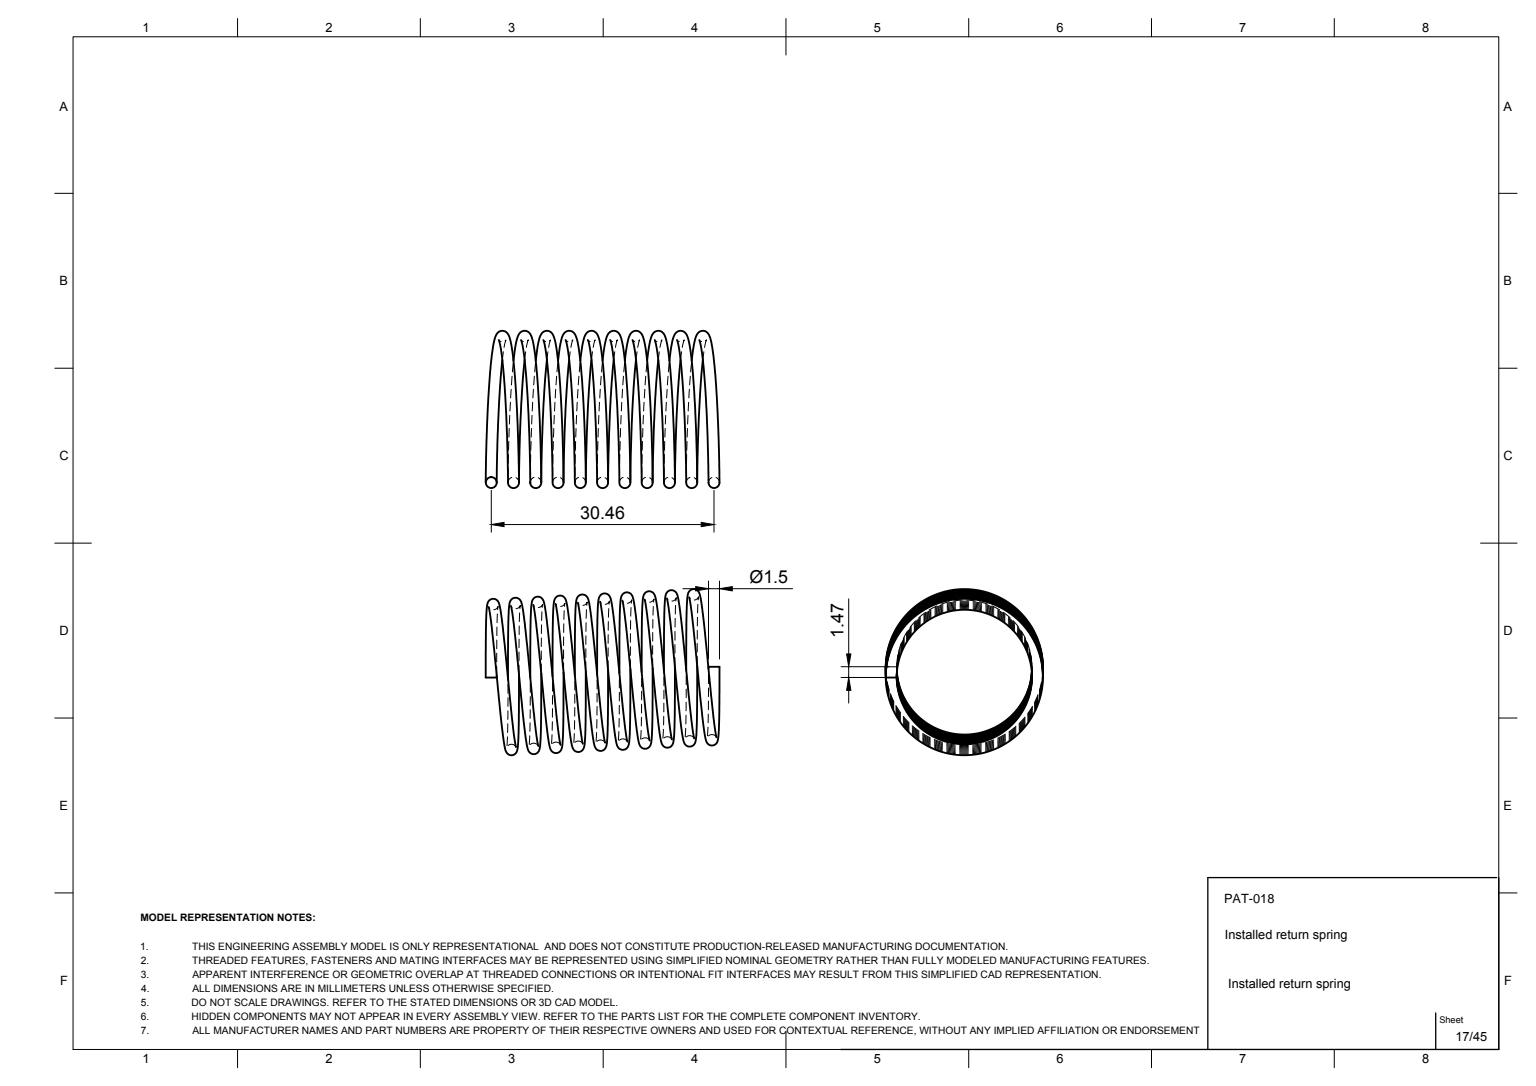
ISO-10303-21;
HEADER;
/* Generated by software containing ST-Developer
 * from STEP Tools, Inc. (www.steptools.com) 
 */

FILE_DESCRIPTION(
/* description */ ('Cam-driven reciprocating slide'),
/* implementation_level */ '2;1');

FILE_NAME(
/* name */ 'Installed return spring.step',
/* time_stamp */ '2026-10-28T03:25:20-07:00',
/* author */ (''),
/* organization */ (''),
/* preprocessor_version */ 'ST-DEVELOPER v20.2',
/* originating_system */ 'Autodesk Translation Framework v15.17.0.0',
/* authorisation */ '');

FILE_SCHEMA (('AUTOMOTIVE_DESIGN { 1 0 10303 214 3 1 1 }'));
ENDSEC;

DATA;
#10=MECHANICAL_DESIGN_GEOMETRIC_PRESENTATION_REPRESENTATION('',(#434),#13277);
#332=B_SPLINE_CURVE_WITH_KNOTS('',3,(#11701,#11702,#11703,#11704,#11705,
#11706,#11707,#11708,#11709,#11710,#11711,#11712,#11713,#11714,#11715,#11716,
#11717,#11718,#11719,#11720,#11721,#11722,#11723,#11724,#11725,#11726,#11727,
#11728,#11729,#11730,#11731,#11732,#11733,#11734,#11735,#11736,#11737,#11738,
#11739,#11740,#11741,#11742,#11743,#11744,#11745,#11746,#11747,#11748,#11749,
#11750,#11751,#11752,#11753,#11754,#11755,#11756,#11757,#11758,#11759,#11760,
#11761,#11762,#11763,#11764,#11765,#11766,#11767,#11768,#11769,#11770,#11771,
#11772,#11773,#11774,#11775,#11776,#11777,#11778,#11779,#11780,#11781,#11782,
#11783,#11784,#11785,#11786,#11787,#11788,#11789,#11790,#11791,#11792,#11793,
#11794,#11795,#11796,#11797,#11798,#11799,#11800,#11801,#11802,#11803,#11804,
#11805,#11806,#11807,#11808,#11809,#11810,#11811,#11812,#11813,#11814,#11815,
#11816,#11817,#11818,#11819,#11820,#11821,#11822,#11823,#11824),
 .UNSPECIFIED.,.F.,.F.,(4,1,1,1,1,1,1,1,1,1,1,1,1,1,1,1,1,1,1,1,1,1,1,1,
1,1,1,1,1,1,1,1,1,1,1,1,1,1,1,1,1,1,1,1,1,1,1,1,1,1,1,1,1,1,1,1,1,1,1,1,
1,1,1,1,1,1,1,1,1,1,1,1,1,1,1,1,1,1,1,1,1,1,1,1,1,1,1,1,1,1,1,1,1,1,1,1,
1,1,1,1,1,1,1,1,1,1,1,1,1,1,1,1,1,1,1,1,1,1,1,1,1,4),(0.,0.00892857142857143,
0.0178571428571429,0.0267857142857143,0.0357142857142857,0.0446428571428571,
0.0535714285714286,0.0625,0.0714285714285714,0.0803571428571428,0.0892857142857143,
0.0982142857142857,0.107142857142857,0.116071428571429,0.125,0.133928571428571,
0.142857142857143,0.150793650793651,0.154761904761905,0.156746031746032,
0.158730158730159,0.166666666666667,0.174603174603175,0.182539682539683,
0.19047619047619,0.202380952380952,0.214285714285714,0.222222222222222,
0.23015873015873,0.238095238095238,0.244047619047619,0.25,0.261904761904762,
0.273809523809524,0.285714285714286,0.297619047619048,0.30952380952381,
0.321428571428571,0.327380952380952,0.333333333333333,0.341269841269841,
0.349206349206349,0.357142857142857,0.365079365079365,0.373015873015873,
0.380952380952381,0.386904761904762,0.392857142857143,0.404761904761905,
0.416666666666667,0.422619047619048,0.428571428571429,0.4375,0.446428571428571,
0.455357142857143,0.464285714285714,0.468253968253968,0.476190476190476,
0.482142857142857,0.488095238095238,0.494047619047619,0.5,0.504464285714286,
0.508928571428571,0.517857142857143,0.526785714285714,0.535714285714286,
0.540178571428571,0.544642857142857,0.553571428571429,0.5625,0.571428571428571,
0.580357142857143,0.589285714285714,0.598214285714286,0.607142857142857,
0.616071428571429,0.625,0.633928571428571,0.642857142857143,0.650793650793651,
0.658730158730159,0.666666666666667,0.672619047619048,0.678571428571428,
0.69047619047619,0.696428571428571,0.702380952380952,0.714285714285714,
0.726190476190476,0.738095238095238,0.746031746031746,0.753968253968254,
0.761904761904762,0.76984126984127,0.777777777777778,0.785714285714286,
0.790178571428571,0.794642857142857,0.803571428571428,0.8125,0.821428571428571,
0.830357142857143,0.839285714285714,0.848214285714286,0.857142857142857,
0.866071428571429,0.875,0.883928571428571,0.892857142857143,0.901785714285714,
0.910714285714286,0.919642857142857,0.928571428571429,0.9375,0.946428571428571,
0.955357142857143,0.964285714285714,0.973214285714286,0.982142857142857,
0.991071428571429,1.),.UNSPECIFIED.);
#347=B_SPLINE_SURFACE_WITH_KNOTS('',3,3,((#10458,#10459,#10460,#10461,#10462,
#10463,#10464,#10465,#10466,#10467,#10468,#10469,#10470,#10471,#10472,#10473,
#10474,#10475,#10476,#10477,#10478,#10479,#10480,#10481,#10482,#10483,#10484,
#10485,#10486,#10487,#10488,#10489,#10490,#10491,#10492,#10493,#10494,#10495,
#10496,#10497,#10498,#10499,#10500,#10501,#10502,#10503,#10504,#10505,#10506,
#10507,#10508,#10509,#10510,#10511,#10512,#10513,#10514,#10515,#10516,#10517,
#10518,#10519,#10520,#10521,#10522,#10523,#10524,#10525,#10526,#10527,#10528,
#10529,#10530,#10531,#10532,#10533,#10534,#10535,#10536,#10537,#10538,#10539,
#10540,#10541,#10542,#10543,#10544,#10545,#10546,#10547,#10548,#10549,#10550,
#10551,#10552,#10553,#10554,#10555,#10556,#10557,#10558,#10559,#10560,#10561,
#10562,#10563,#10564,#10565,#10566,#10567,#10568,#10569,#10570,#10571,#10572,
#10573,#10574,#10575,#10576,#10577,#10578,#10579,#10580,#10581),(#10582,
#10583,#10584,#10585,#10586,#10587,#10588,#10589,#10590,#10591,#10592,#10593,
#10594,#10595,#10596,#10597,#10598,#10599,#10600,#10601,#10602,#10603,#10604,
#10605,#10606,#10607,#10608,#10609,#10610,#10611,#10612,#10613,#10614,#10615,
#10616,#10617,#10618,#10619,#10620,#10621,#10622,#10623,#10624,#10625,#10626,
#10627,#10628,#10629,#10630,#10631,#10632,#10633,#10634,#10635,#10636,#10637,
#10638,#10639,#10640,#10641,#10642,#10643,#10644,#10645,#10646,#10647,#10648,
#10649,#10650,#10651,#10652,#10653,#10654,#10655,#10656,#10657,#10658,#10659,
#10660,#10661,#10662,#10663,#10664,#10665,#10666,#10667,#10668,#10669,#10670,
#10671,#10672,#10673,#10674,#10675,#10676,#10677,#10678,#10679,#10680,#10681,
#10682,#10683,#10684,#10685,#10686,#10687,#10688,#10689,#10690,#10691,#10692,
#10693,#10694,#10695,#10696,#10697,#10698,#10699,#10700,#10701,#10702,#10703,
#10704,#10705),(#10706,#10707,#10708,#10709,#10710,#10711,#10712,#10713,
#10714,#10715,#10716,#10717,#10718,#10719,#10720,#10721,#10722,#10723,#10724,
#10725,#10726,#10727,#10728,#10729,#10730,#10731,#10732,#10733,#10734,#10735,
#10736,#10737,#10738,#10739,#10740,#10741,#10742,#10743,#10744,#10745,#10746,
#10747,#10748,#10749,#10750,#10751,#10752,#10753,#10754,#10755,#10756,#10757,
#10758,#10759,#10760,#10761,#10762,#10763,#10764,#10765,#10766,#10767,#10768,
#10769,#10770,#10771,#10772,#10773,#10774,#10775,#10776,#10777,#10778,#10779,
#10780,#10781,#10782,#10783,#10784,#10785,#10786,#10787,#10788,#10789,#10790,
#10791,#10792,#10793,#10794,#10795,#10796,#10797,#10798,#10799,#10800,#10801,
#10802,#10803,#10804,#10805,#10806,#10807,#10808,#10809,#10810,#10811,#10812,
#10813,#10814,#10815,#10816,#10817,#10818,#10819,#10820,#10821,#10822,#10823,
#10824,#10825,#10826,#10827,#10828,#10829),(#10830,#10831,#10832,#10833,
#10834,#10835,#10836,#10837,#10838,#10839,#10840,#10841,#10842,#10843,#10844,
#10845,#10846,#10847,#10848,#10849,#10850,#10851,#10852,#10853,#10854,#10855,
#10856,#10857,#10858,#10859,#10860,#10861,#10862,#10863,#10864,#10865,#10866,
#10867,#10868,#10869,#10870,#10871,#10872,#10873,#10874,#10875,#10876,#10877,
#10878,#10879,#10880,#10881,#10882,#10883,#10884,#10885,#10886,#10887,#10888,
#10889,#10890,#10891,#10892,#10893,#10894,#10895,#10896,#10897,#10898,#10899,
#10900,#10901,#10902,#10903,#10904,#10905,#10906,#10907,#10908,#10909,#10910,
#10911,#10912,#10913,#10914,#10915,#10916,#10917,#10918,#10919,#10920,#10921,
#10922,#10923,#10924,#10925,#10926,#10927,#10928,#10929,#10930,#10931,#10932,
#10933,#10934,#10935,#10936,#10937,#10938,#10939,#10940,#10941,#10942,#10943,
#10944,#10945,#10946,#10947,#10948,#10949,#10950,#10951,#10952,#10953),
(#10954,#10955,#10956,#10957,#10958,#10959,#10960,#10961,#10962,#10963,
#10964,#10965,#10966,#10967,#10968,#10969,#10970,#10971,#10972,#10973,#10974,
#10975,#10976,#10977,#10978,#10979,#10980,#10981,#10982,#10983,#10984,#10985,
#10986,#10987,#10988,#10989,#10990,#10991,#10992,#10993,#10994,#10995,#10996,
#10997,#10998,#10999,#11000,#11001,#11002,#11003,#11004,#11005,#11006,#11007,
#11008,#11009,#11010,#11011,#11012,#11013,#11014,#11015,#11016,#11017,#11018,
#11019,#11020,#11021,#11022,#11023,#11024,#11025,#11026,#11027,#11028,#11029,
#11030,#11031,#11032,#11033,#11034,#11035,#11036,#11037,#11038,#11039,#11040,
#11041,#11042,#11043,#11044,#11045,#11046,#11047,#11048,#11049,#11050,#11051,
#11052,#11053,#11054,#11055,#11056,#11057,#11058,#11059,#11060,#11061,#11062,
#11063,#11064,#11065,#11066,#11067,#11068,#11069,#11070,#11071,#11072,#11073,
#11074,#11075,#11076,#11077),(#11078,#11079,#11080,#11081,#11082,#11083,
#11084,#11085,#11086,#11087,#11088,#11089,#11090,#11091,#11092,#11093,#11094,
#11095,#11096,#11097,#11098,#11099,#11100,#11101,#11102,#11103,#11104,#11105,
#11106,#11107,#11108,#11109,#11110,#11111,#11112,#11113,#11114,#11115,#11116,
#11117,#11118,#11119,#11120,#11121,#11122,#11123,#11124,#11125,#11126,#11127,
#11128,#11129,#11130,#11131,#11132,#11133,#11134,#11135,#11136,#11137,#11138,
#11139,#11140,#11141,#11142,#11143,#11144,#11145,#11146,#11147,#11148,#11149,
#11150,#11151,#11152,#11153,#11154,#11155,#11156,#11157,#11158,#11159,#11160,
#11161,#11162,#11163,#11164,#11165,#11166,#11167,#11168,#11169,#11170,#11171,
#11172,#11173,#11174,#11175,#11176,#11177,#11178,#11179,#11180,#11181,#11182,
#11183,#11184,#11185,#11186,#11187,#11188,#11189,#11190,#11191,#11192,#11193,
#11194,#11195,#11196,#11197,#11198,#11199,#11200,#11201),(#11202,#11203,
#11204,#11205,#11206,#11207,#11208,#11209,#11210,#11211,#11212,#11213,#11214,
#11215,#11216,#11217,#11218,#11219,#11220,#11221,#11222,#11223,#11224,#11225,
#11226,#11227,#11228,#11229,#11230,#11231,#11232,#11233,#11234,#11235,#11236,
#11237,#11238,#11239,#11240,#11241,#11242,#11243,#11244,#11245,#11246,#11247,
#11248,#11249,#11250,#11251,#11252,#11253,#11254,#11255,#11256,#11257,#11258,
#11259,#11260,#11261,#11262,#11263,#11264,#11265,#11266,#11267,#11268,#11269,
#11270,#11271,#11272,#11273,#11274,#11275,#11276,#11277,#11278,#11279,#11280,
#11281,#11282,#11283,#11284,#11285,#11286,#11287,#11288,#11289,#11290,#11291,
#11292,#11293,#11294,#11295,#11296,#11297,#11298,#11299,#11300,#11301,#11302,
#11303,#11304,#11305,#11306,#11307,#11308,#11309,#11310,#11311,#11312,#11313,
#11314,#11315,#11316,#11317,#11318,#11319,#11320,#11321,#11322,#11323,#11324,
#11325),(#11326,#11327,#11328,#11329,#11330,#11331,#11332,#11333,#11334,
#11335,#11336,#11337,#11338,#11339,#11340,#11341,#11342,#11343,#11344,#11345,
#11346,#11347,#11348,#11349,#11350,#11351,#11352,#11353,#11354,#11355,#11356,
#11357,#11358,#11359,#11360,#11361,#11362,#11363,#11364,#11365,#11366,#11367,
#11368,#11369,#11370,#11371,#11372,#11373,#11374,#11375,#11376,#11377,#11378,
#11379,#11380,#11381,#11382,#11383,#11384,#11385,#11386,#11387,#11388,#11389,
#11390,#11391,#11392,#11393,#11394,#11395,#11396,#11397,#11398,#11399,#11400,
#11401,#11402,#11403,#11404,#11405,#11406,#11407,#11408,#11409,#11410,#11411,
#11412,#11413,#11414,#11415,#11416,#11417,#11418,#11419,#11420,#11421,#11422,
#11423,#11424,#11425,#11426,#11427,#11428,#11429,#11430,#11431,#11432,#11433,
#11434,#11435,#11436,#11437,#11438,#11439,#11440,#11441,#11442,#11443,#11444,
#11445,#11446,#11447,#11448,#11449),(#11450,#11451,#11452,#11453,#11454,
#11455,#11456,#11457,#11458,#11459,#11460,#11461,#11462,#11463,#11464,#11465,
#11466,#11467,#11468,#11469,#11470,#11471,#11472,#11473,#11474,#11475,#11476,
#11477,#11478,#11479,#11480,#11481,#11482,#11483,#11484,#11485,#11486,#11487,
#11488,#11489,#11490,#11491,#11492,#11493,#11494,#11495,#11496,#11497,#11498,
#11499,#11500,#11501,#11502,#11503,#11504,#11505,#11506,#11507,#11508,#11509,
#11510,#11511,#11512,#11513,#11514,#11515,#11516,#11517,#11518,#11519,#11520,
#11521,#11522,#11523,#11524,#11525,#11526,#11527,#11528,#11529,#11530,#11531,
#11532,#11533,#11534,#11535,#11536,#11537,#11538,#11539,#11540,#11541,#11542,
#11543,#11544,#11545,#11546,#11547,#11548,#11549,#11550,#11551,#11552,#11553,
#11554,#11555,#11556,#11557,#11558,#11559,#11560,#11561,#11562,#11563,#11564,
#11565,#11566,#11567,#11568,#11569,#11570,#11571,#11572,#11573),(#11574,
#11575,#11576,#11577,#11578,#11579,#11580,#11581,#11582,#11583,#11584,#11585,
#11586,#11587,#11588,#11589,#11590,#11591,#11592,#11593,#11594,#11595,#11596,
#11597,#11598,#11599,#11600,#11601,#11602,#11603,#11604,#11605,#11606,#11607,
#11608,#11609,#11610,#11611,#11612,#11613,#11614,#11615,#11616,#11617,#11618,
#11619,#11620,#11621,#11622,#11623,#11624,#11625,#11626,#11627,#11628,#11629,
#11630,#11631,#11632,#11633,#11634,#11635,#11636,#11637,#11638,#11639,#11640,
#11641,#11642,#11643,#11644,#11645,#11646,#11647,#11648,#11649,#11650,#11651,
#11652,#11653,#11654,#11655,#11656,#11657,#11658,#11659,#11660,#11661,#11662,
#11663,#11664,#11665,#11666,#11667,#11668,#11669,#11670,#11671,#11672,#11673,
#11674,#11675,#11676,#11677,#11678,#11679,#11680,#11681,#11682,#11683,#11684,
#11685,#11686,#11687,#11688,#11689,#11690,#11691,#11692,#11693,#11694,#11695,
#11696,#11697)),.UNSPECIFIED.,.T.,.F.,.F.,(4,1,1,1,1,1,1,4),(4,1,1,1,1,
1,1,1,1,1,1,1,1,1,1,1,1,1,1,1,1,1,1,1,1,1,1,1,1,1,1,1,1,1,1,1,1,1,1,1,1,
1,1,1,1,1,1,1,1,1,1,1,1,1,1,1,1,1,1,1,1,1,1,1,1,1,1,1,1,1,1,1,1,1,1,1,1,
1,1,1,1,1,1,1,1,1,1,1,1,1,1,1,1,1,1,1,1,1,1,1,1,1,1,1,1,1,1,1,1,1,1,1,1,
1,1,1,1,1,1,1,1,4),(-3.14159265358979,-2.24399475256414,-1.34639685153848,
-0.448798950512828,0.448798950512828,1.34639685153848,2.24399475256414,
3.14159265358979),(0.,0.00892857142857143,0.0178571428571429,0.0267857142857143,
0.0357142857142857,0.0446428571428571,0.0535714285714286,0.0625,0.0714285714285714,
0.0803571428571428,0.0892857142857143,0.0982142857142857,0.107142857142857,
0.116071428571429,0.125,0.133928571428571,0.142857142857143,0.150793650793651,
0.154761904761905,0.156746031746032,0.158730158730159,0.166666666666667,
0.174603174603175,0.182539682539683,0.19047619047619,0.202380952380952,
0.214285714285714,0.222222222222222,0.23015873015873,0.238095238095238,
0.244047619047619,0.25,0.261904761904762,0.273809523809524,0.285714285714286,
0.297619047619048,0.30952380952381,0.321428571428571,0.327380952380952,
0.333333333333333,0.341269841269841,0.349206349206349,0.357142857142857,
0.365079365079365,0.373015873015873,0.380952380952381,0.386904761904762,
0.392857142857143,0.404761904761905,0.416666666666667,0.422619047619048,
0.428571428571429,0.4375,0.446428571428571,0.455357142857143,0.464285714285714,
0.468253968253968,0.476190476190476,0.482142857142857,0.488095238095238,
0.494047619047619,0.5,0.504464285714286,0.508928571428571,0.517857142857143,
0.526785714285714,0.535714285714286,0.540178571428571,0.544642857142857,
0.553571428571429,0.5625,0.571428571428571,0.580357142857143,0.589285714285714,
0.598214285714286,0.607142857142857,0.616071428571429,0.625,0.633928571428571,
0.642857142857143,0.650793650793651,0.658730158730159,0.666666666666667,
0.672619047619048,0.678571428571428,0.69047619047619,0.696428571428571,
0.702380952380952,0.714285714285714,0.726190476190476,0.738095238095238,
0.746031746031746,0.753968253968254,0.761904761904762,0.76984126984127,
0.777777777777778,0.785714285714286,0.790178571428571,0.794642857142857,
0.803571428571428,0.8125,0.821428571428571,0.830357142857143,0.839285714285714,
0.848214285714286,0.857142857142857,0.866071428571429,0.875,0.883928571428571,
0.892857142857143,0.901785714285714,0.910714285714286,0.919642857142857,
0.928571428571429,0.9375,0.946428571428571,0.955357142857143,0.964285714285714,
0.973214285714286,0.982142857142857,0.991071428571429,1.),.UNSPECIFIED.);
#360=SHAPE_REPRESENTATION_RELATIONSHIP('SRR','None',#13453,#397);
#397=ADVANCED_BREP_SHAPE_REPRESENTATION('',(#478),#13248);
#434=STYLED_ITEM('',(#13720),#478);
#478=MANIFOLD_SOLID_BREP('Body1',#6410);
#762=PLANE('',#7152);
#763=PLANE('',#7153);
#1049=FACE_OUTER_BOUND('',#1539,.T.);
#1050=FACE_OUTER_BOUND('',#1540,.T.);
#1051=FACE_OUTER_BOUND('',#1541,.T.);
#1539=EDGE_LOOP('',(#5002,#5003,#5004,#5005));
#1540=EDGE_LOOP('',(#5006));
#1541=EDGE_LOOP('',(#5007));
#2845=CIRCLE('',#7150,0.075);
#2846=CIRCLE('',#7151,0.075);
#3257=VERTEX_POINT('',#11698);
#3258=VERTEX_POINT('',#11700);
#3891=EDGE_CURVE('',#3257,#3257,#2845,.T.);
#3892=EDGE_CURVE('',#3257,#3258,#332,.T.);
#3893=EDGE_CURVE('',#3258,#3258,#2846,.T.);
#5002=ORIENTED_EDGE('',*,*,#3891,.T.);
#5003=ORIENTED_EDGE('',*,*,#3892,.T.);
#5004=ORIENTED_EDGE('',*,*,#3893,.F.);
#5005=ORIENTED_EDGE('',*,*,#3892,.F.);
#5006=ORIENTED_EDGE('',*,*,#3893,.T.);
#5007=ORIENTED_EDGE('',*,*,#3891,.F.);
#6167=ADVANCED_FACE('',(#1049),#347,.T.);
#6168=ADVANCED_FACE('',(#1050),#762,.T.);
#6169=ADVANCED_FACE('',(#1051),#763,.F.);
#6410=CLOSED_SHELL('',(#6167,#6168,#6169));
#7149=AXIS2_PLACEMENT_3D('',#10457,#8460,#8461);
#7150=AXIS2_PLACEMENT_3D('',#11699,#8462,#8463);
#7151=AXIS2_PLACEMENT_3D('',#11825,#8464,#8465);
#7152=AXIS2_PLACEMENT_3D('',#11826,#8466,#8467);
#7153=AXIS2_PLACEMENT_3D('',#11827,#8468,#8469);
#8460=DIRECTION('axis',(0.,0.,1.));
#8461=DIRECTION('refdir',(1.,0.,0.));
#8462=DIRECTION('center_axis',(-0.000134463754131944,0.998830887797922,
0.0483408678067963));
#8463=DIRECTION('ref_axis',(6.50770273904549E-6,-0.0483408673687592,0.998830896848754));
#8464=DIRECTION('center_axis',(0.000134463742439319,0.998830887795465,0.0483408678575998));
#8465=DIRECTION('ref_axis',(-0.0950425701692232,0.0481348041224881,-0.994308780252753));
#8466=DIRECTION('center_axis',(0.000134463742439319,0.998830887795465,0.0483408678575998));
#8467=DIRECTION('ref_axis',(-0.0950425701692232,0.0481348041224881,-0.994308780252753));
#8468=DIRECTION('center_axis',(-0.000134463754131944,0.998830887797922,
0.0483408678067963));
#8469=DIRECTION('ref_axis',(6.50770273904549E-6,-0.0483408673687592,0.998830896848754));
#10457=CARTESIAN_POINT('',(0.,0.,0.));
#10458=CARTESIAN_POINT('Ctrl Pts',(0.999999511922295,0.00362556505265694,
7.80008768273634));
#10459=CARTESIAN_POINT('Ctrl Pts',(0.999974254701651,0.191242609375982,
7.80916786923111));
#10460=CARTESIAN_POINT('Ctrl Pts',(0.892341067491657,0.564938782877452,
7.82733932423682));
#10461=CARTESIAN_POINT('Ctrl Pts',(0.456009237357814,0.955278731473674,
7.85465504855182));
#10462=CARTESIAN_POINT('Ctrl Pts',(-0.122182810478375,1.05350592491678,
7.88202502929242));
#10463=CARTESIAN_POINT('Ctrl Pts',(-0.665220911419956,0.828753483606749,
7.90945086692426));
#10464=CARTESIAN_POINT('Ctrl Pts',(-1.00612665101876,0.348504727673495,
7.93693161942117));
#10465=CARTESIAN_POINT('Ctrl Pts',(-1.03937057711115,-0.24065277058934,
7.96446742990799));
#10466=CARTESIAN_POINT('Ctrl Pts',(-0.753506480379588,-0.758233234780652,
7.99205790686499));
#10467=CARTESIAN_POINT('Ctrl Pts',(-0.23507859765888,-1.04495072049649,
8.01970284677932));
#10468=CARTESIAN_POINT('Ctrl Pts',(0.357583215672993,-1.01183827364816,
8.04740190675199));
#10469=CARTESIAN_POINT('Ctrl Pts',(0.842723866190013,-0.667819008067397,
8.07515475263842));
#10470=CARTESIAN_POINT('Ctrl Pts',(1.07090748459127,-0.117361728527591,
8.1029609908626));
#10471=CARTESIAN_POINT('Ctrl Pts',(0.971068313490196,0.471237645030074,
8.13082019638131));
#10472=CARTESIAN_POINT('Ctrl Pts',(0.572615291983895,0.917345600069376,
8.15873190469605));
#10473=CARTESIAN_POINT('Ctrl Pts',(-0.00315068596155565,1.08336827030711,
8.18669561143439));
#10474=CARTESIAN_POINT('Ctrl Pts',(-0.580114085036881,0.917350780124834,
8.21471077684478));
#10475=CARTESIAN_POINT('Ctrl Pts',(-0.966051395769627,0.48549839913134,
8.24173733490367));
#10476=CARTESIAN_POINT('Ctrl Pts',(-1.05781582749726,0.0299567596628159,
8.2636033984339));
#10477=CARTESIAN_POINT('Ctrl Pts',(-1.00496213983024,-0.268439331682945,
8.27819794787177));
#10478=CARTESIAN_POINT('Ctrl Pts',(-0.94403781713285,-0.429519542479439,
8.28654256698954));
#10479=CARTESIAN_POINT('Ctrl Pts',(-0.823382078993268,-0.658140969899007,
8.29906435736913));
#10480=CARTESIAN_POINT('Ctrl Pts',(-0.537625296367964,-0.93706913925231,
8.31786521711992));
#10481=CARTESIAN_POINT('Ctrl Pts',(-0.0238288726443125,-1.08214769701979,
8.34297130007593));
#10482=CARTESIAN_POINT('Ctrl Pts',(0.496636287796273,-0.96271505408145,
8.36811512451513));
#10483=CARTESIAN_POINT('Ctrl Pts',(0.966152438091784,-0.550650417462692,
8.39749297986939));
#10484=CARTESIAN_POINT('Ctrl Pts',(1.13301488484768,0.17354695961988,8.43112871623582));
#10485=CARTESIAN_POINT('Ctrl Pts',(0.759782029367692,0.81792928250629,8.46483592073065));
#10486=CARTESIAN_POINT('Ctrl Pts',(0.18659690053678,1.07520238454981,8.49438045894607));
#10487=CARTESIAN_POINT('Ctrl Pts',(-0.350443601960556,1.03519669411318,
8.51973848476555));
#10488=CARTESIAN_POINT('Ctrl Pts',(-0.766297161890012,0.766560498033478,
8.54301401492018));
#10489=CARTESIAN_POINT('Ctrl Pts',(-1.00188555557132,0.390501874334262,
8.56419748306598));
#10490=CARTESIAN_POINT('Ctrl Pts',(-1.10276576842174,-0.133757727725488,
8.5896418232172));
#10491=CARTESIAN_POINT('Ctrl Pts',(-0.847050948528023,-0.7885712029239,
8.6214918164511));
#10492=CARTESIAN_POINT('Ctrl Pts',(-0.0842079511184448,-1.15633714773807,
8.65978061793639));
#10493=CARTESIAN_POINT('Ctrl Pts',(0.72557322963091,-0.906499072035091,
8.69813561803015));
#10494=CARTESIAN_POINT('Ctrl Pts',(1.15047751535783,-0.171671665185466,
8.73655413319947));
#10495=CARTESIAN_POINT('Ctrl Pts',(0.961273159473049,0.658124915791643,
8.77503338584849));
#10496=CARTESIAN_POINT('Ctrl Pts',(0.375126711265494,1.05675920723847,8.80714766479813));
#10497=CARTESIAN_POINT('Ctrl Pts',(-0.164183045710825,1.07538023554299,
8.8328665668906));
#10498=CARTESIAN_POINT('Ctrl Pts',(-0.588587403918608,0.927569264768944,
8.85431383603483));
#10499=CARTESIAN_POINT('Ctrl Pts',(-0.947989492545562,0.577208917394653,
8.87792434906622));
#10500=CARTESIAN_POINT('Ctrl Pts',(-1.10961450093061,0.0536146968196933,
8.90370345540594));
#10501=CARTESIAN_POINT('Ctrl Pts',(-1.00082022593385,-0.483727092204472,
8.92950382341385));
#10502=CARTESIAN_POINT('Ctrl Pts',(-0.648169490504554,-0.904286310022195,
8.95532452406706));
#10503=CARTESIAN_POINT('Ctrl Pts',(-0.137073525470092,-1.1047399934849,
8.98116461266558));
#10504=CARTESIAN_POINT('Ctrl Pts',(0.362995552358674,-1.04213062048012,
9.0048682588092));
#10505=CARTESIAN_POINT('Ctrl Pts',(0.744903368537152,-0.801138176501351,
9.02642976126975));
#10506=CARTESIAN_POINT('Ctrl Pts',(1.06927029269131,-0.365389501861442,
9.05231612054031));
#10507=CARTESIAN_POINT('Ctrl Pts',(1.12442623960627,0.347295239484755,9.08469656290588));
#10508=CARTESIAN_POINT('Ctrl Pts',(0.676375081319218,0.906916376424927,
9.11710422215215));
#10509=CARTESIAN_POINT('Ctrl Pts',(0.162505682592346,1.08489901523682,9.14304497362832));
#10510=CARTESIAN_POINT('Ctrl Pts',(-0.313134592199748,1.06806757295122,
9.16575116654966));
#10511=CARTESIAN_POINT('Ctrl Pts',(-0.80020652042605,0.79906113083438,9.19171186155256));
#10512=CARTESIAN_POINT('Ctrl Pts',(-1.1030130064212,0.251155630516143,9.22093071361268));
#10513=CARTESIAN_POINT('Ctrl Pts',(-1.06806000491819,-0.374587327913118,
9.25016115867103));
#10514=CARTESIAN_POINT('Ctrl Pts',(-0.772382685892504,-0.790331103336901,
9.27398680631869));
#10515=CARTESIAN_POINT('Ctrl Pts',(-0.369190625906315,-1.03674084848642,
9.29673431868371));
#10516=CARTESIAN_POINT('Ctrl Pts',(0.038576143908095,-1.10885924555696,
9.31623572825941));
#10517=CARTESIAN_POINT('Ctrl Pts',(0.477637122556786,-0.990697811322314,
9.33790778885712));
#10518=CARTESIAN_POINT('Ctrl Pts',(0.806650901305872,-0.74814670656117,
9.35741515109002));
#10519=CARTESIAN_POINT('Ctrl Pts',(1.02427838601106,-0.401712335365787,
9.37692457700679));
#10520=CARTESIAN_POINT('Ctrl Pts',(1.0939769734331,-0.0333100781542004,
9.39480970049716));
#10521=CARTESIAN_POINT('Ctrl Pts',(1.04649131988823,0.301575311206996,9.4110697587252));
#10522=CARTESIAN_POINT('Ctrl Pts',(0.881091959620118,0.67241835967004,9.43058245602211));
#10523=CARTESIAN_POINT('Ctrl Pts',(0.491781434765328,1.02078793932956,9.45497403322699));
#10524=CARTESIAN_POINT('Ctrl Pts',(-0.12690622562046,1.12590240218231,9.48424354952418));
#10525=CARTESIAN_POINT('Ctrl Pts',(-0.609455917268022,0.925702271760676,
9.50863324396813));
#10526=CARTESIAN_POINT('Ctrl Pts',(-0.887901221690915,0.630308788370616,
9.52814330365954));
#10527=CARTESIAN_POINT('Ctrl Pts',(-1.07473168029324,0.269973249594665,
9.54765198252425));
#10528=CARTESIAN_POINT('Ctrl Pts',(-1.10429179277937,-0.251571030257534,
9.57203477138778));
#10529=CARTESIAN_POINT('Ctrl Pts',(-0.800909981683876,-0.800300061810875,
9.60128772802457));
#10530=CARTESIAN_POINT('Ctrl Pts',(-0.252449360054481,-1.10339503360944,
9.63053279474191));
#10531=CARTESIAN_POINT('Ctrl Pts',(0.373097965965379,-1.06824993186655,
9.65976848374119));
#10532=CARTESIAN_POINT('Ctrl Pts',(0.883833752107615,-0.705802685092957,
9.68899331286683));
#10533=CARTESIAN_POINT('Ctrl Pts',(1.12336062251109,-0.127424704798401,
9.71820580950298));
#10534=CARTESIAN_POINT('Ctrl Pts',(1.01851100341375,0.489451283507362,9.7474045069875));
#10535=CARTESIAN_POINT('Ctrl Pts',(0.601719134479875,0.955745657723928,
9.7765879476835));
#10536=CARTESIAN_POINT('Ctrl Pts',(0.00114764771726767,1.12873118183179,
9.80575469579441));
#10537=CARTESIAN_POINT('Ctrl Pts',(-0.599201162150444,0.955775323307818,
9.83490331154648));
#10538=CARTESIAN_POINT('Ctrl Pts',(-0.999441525170258,0.507519999720283,
9.86295352909998));
#10539=CARTESIAN_POINT('Ctrl Pts',(-1.11281367201976,-0.0541281101275826,
9.88990656850941));
#10540=CARTESIAN_POINT('Ctrl Pts',(-0.950656776962806,-0.578991698652294,
9.91576396161208));
#10541=CARTESIAN_POINT('Ctrl Pts',(-0.590339529048702,-0.930637197709755,
9.93944961788225));
#10542=CARTESIAN_POINT('Ctrl Pts',(-0.164606104863989,-1.07875415066616,
9.96096785470298));
#10543=CARTESIAN_POINT('Ctrl Pts',(0.376774813272184,-1.06001813820014,
9.98677462212391));
#10544=CARTESIAN_POINT('Ctrl Pts',(0.846936223245377,-0.740877146125449,
10.0125579187175));
#10545=CARTESIAN_POINT('Ctrl Pts',(1.06107082068352,-0.244205647020787,
10.0383162020965));
#10546=CARTESIAN_POINT('Ctrl Pts',(1.08304241869915,0.294959566025181,10.0640572896683));
#10547=CARTESIAN_POINT('Ctrl Pts',(0.729014765427379,0.91016891175548,10.0962004771028));
#10548=CARTESIAN_POINT('Ctrl Pts',(-0.0857101331349617,1.16113591721249,
10.1347162317012));
#10549=CARTESIAN_POINT('Ctrl Pts',(-0.764643776951617,0.832591967114145,
10.1689000478027));
#10550=CARTESIAN_POINT('Ctrl Pts',(-1.0674640769428,0.273793097090764,10.1987708394967));
#10551=CARTESIAN_POINT('Ctrl Pts',(-1.06731019456222,-0.269314357950732,
10.22434609796));
#10552=CARTESIAN_POINT('Ctrl Pts',(-0.807788715964582,-0.746430097707613,
10.2498922819076));
#10553=CARTESIAN_POINT('Ctrl Pts',(-0.352065023972404,-1.04036411773073,
10.275408603128));
#10554=CARTESIAN_POINT('Ctrl Pts',(0.18806187608402,-1.08063605589285,10.3008942987819));
#10555=CARTESIAN_POINT('Ctrl Pts',(0.609132779330515,-0.890423751871434,
10.3226365334534));
#10556=CARTESIAN_POINT('Ctrl Pts',(0.866237924373777,-0.61783839929423,
10.3406489137734));
#10557=CARTESIAN_POINT('Ctrl Pts',(1.04872505851243,-0.26577216648544,10.3597071335657));
#10558=CARTESIAN_POINT('Ctrl Pts',(1.07750116603121,0.243190015038482,10.3835038803323));
#10559=CARTESIAN_POINT('Ctrl Pts',(0.781688530878207,0.777999980609408,
10.4120173608425));
#10560=CARTESIAN_POINT('Ctrl Pts',(0.247719136142376,1.07295015546241,10.4404872688827));
#10561=CARTESIAN_POINT('Ctrl Pts',(-0.360486616831365,1.03867188015668,
10.4689126947258));
#10562=CARTESIAN_POINT('Ctrl Pts',(-0.856395421979649,0.686612064758622,
10.4972927514314));
#10563=CARTESIAN_POINT('Ctrl Pts',(-1.08862861454113,0.125592182065228,
10.5256265935356));
#10564=CARTESIAN_POINT('Ctrl Pts',(-0.986944606168628,-0.472001059894419,
10.5539134034074));
#10565=CARTESIAN_POINT('Ctrl Pts',(-0.583594151562567,-0.923132799570535,
10.5821523997639));
#10566=CARTESIAN_POINT('Ctrl Pts',(-0.00304950196324622,-1.09023227406354,
10.6103428416619));
#10567=CARTESIAN_POINT('Ctrl Pts',(0.576397100829433,-0.923141572582211,
10.6384840153271));
#10568=CARTESIAN_POINT('Ctrl Pts',(0.977415745977647,-0.474174920735025,
10.666575250779));
#10569=CARTESIAN_POINT('Ctrl Pts',(1.07791854333959,0.118262177227866,10.6946159100158));
#10570=CARTESIAN_POINT('Ctrl Pts',(0.848237687346995,0.672348815808936,
10.7226053954193));
#10571=CARTESIAN_POINT('Ctrl Pts',(0.35987034323251,1.01866632704243,10.750543145368));
#10572=CARTESIAN_POINT('Ctrl Pts',(-0.23677931351889,1.05200727853759,10.7784286311663));
#10573=CARTESIAN_POINT('Ctrl Pts',(-0.758730842080508,0.763346883548158,
10.8062613781485));
#10574=CARTESIAN_POINT('Ctrl Pts',(-1.04655744183574,0.242222537004657,
10.8340409125563));
#10575=CARTESIAN_POINT('Ctrl Pts',(-1.01308793288556,-0.351003613269005,
10.8617668734456));
#10576=CARTESIAN_POINT('Ctrl Pts',(-0.669814425530371,-0.834593746223134,
10.889438771651));
#10577=CARTESIAN_POINT('Ctrl Pts',(-0.122977155730889,-1.06092281666227,
10.9170565165848));
#10578=CARTESIAN_POINT('Ctrl Pts',(0.459284142389985,-0.962004532278344,
10.9446192376113));
#10579=CARTESIAN_POINT('Ctrl Pts',(0.898703292351648,-0.568910379520766,
10.9721279252064));
#10580=CARTESIAN_POINT('Ctrl Pts',(1.0071027576084,-0.192548907318078,10.9904290025552));
#10581=CARTESIAN_POINT('Ctrl Pts',(1.00712819276269,-0.00361011030918905,
10.999573158519));
#10582=CARTESIAN_POINT('Ctrl Pts',(0.977559564599991,0.00362254416133655,
7.80008768273634));
#10583=CARTESIAN_POINT('Ctrl Pts',(0.977534866689631,0.18708488976632,7.80896679240822));
#10584=CARTESIAN_POINT('Ctrl Pts',(0.872322415557346,0.552393922726298,
7.82672927903241));
#10585=CARTESIAN_POINT('Ctrl Pts',(0.445718486862071,0.934060193527018,
7.85343643021417));
#10586=CARTESIAN_POINT('Ctrl Pts',(-0.119636647243807,1.03010841597759,
7.88019745241192));
#10587=CARTESIAN_POINT('Ctrl Pts',(-0.650678967970242,0.810334582562273,
7.90701638678188));
#10588=CARTESIAN_POINT('Ctrl Pts',(-0.984099810756226,0.340647684643633,
7.93389180692065));
#10589=CARTESIAN_POINT('Ctrl Pts',(-1.01663027186777,-0.235634070049338,
7.96082469172386));
#10590=CARTESIAN_POINT('Ctrl Pts',(-0.736984385597307,-0.741986536865251,
7.98781490109356));
#10591=CARTESIAN_POINT('Ctrl Pts',(-0.229735381724658,-1.02253990905577,
8.01486274772683));
#10592=CARTESIAN_POINT('Ctrl Pts',(0.350260356893508,-0.990152762857837,
8.04196828714851));
#10593=CARTESIAN_POINT('Ctrl Pts',(0.825134997145517,-0.653436415065432,
8.06913163396793));
#10594=CARTESIAN_POINT('Ctrl Pts',(1.04855042623966,-0.114534980319938,
8.0963528116897));
#10595=CARTESIAN_POINT('Ctrl Pts',(0.950805881040683,0.461848534559346,
8.12363183217922));
#10596=CARTESIAN_POINT('Ctrl Pts',(0.560550547543524,0.89881493391695,8.15096862326752));
#10597=CARTESIAN_POINT('Ctrl Pts',(-0.00352941556499671,1.06149499328244,
8.17836313496341));
#10598=CARTESIAN_POINT('Ctrl Pts',(-0.568945432596404,0.898829335752363,
8.2058151151295));
#10599=CARTESIAN_POINT('Ctrl Pts',(-0.947276485604154,0.475525661597343,
8.23230571210832));
#10600=CARTESIAN_POINT('Ctrl Pts',(-1.03726714683262,0.0288659729588981,
8.25374377338214));
#10601=CARTESIAN_POINT('Ctrl Pts',(-0.985433969276193,-0.263782787095173,
8.26805657036754));
#10602=CARTESIAN_POINT('Ctrl Pts',(-0.925676430299761,-0.421778753641079,
8.27624126130311));
#10603=CARTESIAN_POINT('Ctrl Pts',(-0.807324773446438,-0.646038667836079,
8.28852379480006));
#10604=CARTESIAN_POINT('Ctrl Pts',(-0.526999308588214,-0.919685240659636,
8.30696610050169));
#10605=CARTESIAN_POINT('Ctrl Pts',(-0.0227868718866388,-1.06208690811312,
8.33160304885951));
#10606=CARTESIAN_POINT('Ctrl Pts',(0.48813066286185,-0.944858682751246,
8.35628380467876));
#10607=CARTESIAN_POINT('Ctrl Pts',(0.949193206679585,-0.540258543297488,
8.38512932713425));
#10608=CARTESIAN_POINT('Ctrl Pts',(1.11316501047521,0.171118961858805,8.41816585508126));
#10609=CARTESIAN_POINT('Ctrl Pts',(0.746415595315959,0.80445351686326,8.45128858999103));
#10610=CARTESIAN_POINT('Ctrl Pts',(0.18282724257968,1.05745094591858,8.48033697773421));
#10611=CARTESIAN_POINT('Ctrl Pts',(-0.345419524449013,1.01812107532715,
8.50527861143673));
#10612=CARTESIAN_POINT('Ctrl Pts',(-0.754611477987093,0.753819380993674,
8.52817815885987));
#10613=CARTESIAN_POINT('Ctrl Pts',(-0.986508596508495,0.383672790215633,
8.54902745839679));
#10614=CARTESIAN_POINT('Ctrl Pts',(-1.08584686716394,-0.132493523343181,
8.57407782842635));
#10615=CARTESIAN_POINT('Ctrl Pts',(-0.834046887505374,-0.777476644629888,
8.60544368069453));
#10616=CARTESIAN_POINT('Ctrl Pts',(-0.0822626488291713,-1.14001853467866,
8.64317523263573));
#10617=CARTESIAN_POINT('Ctrl Pts',(0.716337570524463,-0.893726913198842,
8.68099425934154));
#10618=CARTESIAN_POINT('Ctrl Pts',(1.13571087813116,-0.168674579522828,
8.71889923674692));
#10619=CARTESIAN_POINT('Ctrl Pts',(0.94899413688568,0.65068751575287,8.75688888882341));
#10620=CARTESIAN_POINT('Ctrl Pts',(0.369924963489578,1.04461917501135,8.78861243968945));
#10621=CARTESIAN_POINT('Ctrl Pts',(-0.163212573764178,1.06304769871494,
8.81403513535945));
#10622=CARTESIAN_POINT('Ctrl Pts',(-0.582898835599307,0.916898919717624,
8.83524177562921));
#10623=CARTESIAN_POINT('Ctrl Pts',(-0.938452485791775,0.570332830031077,
8.8585957898151));
#10624=CARTESIAN_POINT('Ctrl Pts',(-1.098449244479,0.0521610218923669,8.88410456256871));
#10625=CARTESIAN_POINT('Ctrl Pts',(-0.990747044809017,-0.479905179357058,
8.9096503715829));
#10626=CARTESIAN_POINT('Ctrl Pts',(-0.641456339423732,-0.89652388800662,
8.93522327648824));
#10627=CARTESIAN_POINT('Ctrl Pts',(-0.134922280861396,-1.09521608917999,
8.96083178186041));
#10628=CARTESIAN_POINT('Ctrl Pts',(0.360901232907297,-1.03317015380971,
8.98433058053565));
#10629=CARTESIAN_POINT('Ctrl Pts',(0.739743448699196,-0.794125607724712,
9.00571660323141));
#10630=CARTESIAN_POINT('Ctrl Pts',(1.06162643141654,-0.361743804765045,
9.03140126883326));
#10631=CARTESIAN_POINT('Ctrl Pts',(1.11648086851777,0.345841238273162,9.06354866838759));
#10632=CARTESIAN_POINT('Ctrl Pts',(0.671412092383133,0.901879124054754,
9.09573676847456));
#10633=CARTESIAN_POINT('Ctrl Pts',(0.160560298699368,1.07883883046449,9.12152345956742));
#10634=CARTESIAN_POINT('Ctrl Pts',(-0.31245850549709,1.06211512228001,9.14410225952631));
#10635=CARTESIAN_POINT('Ctrl Pts',(-0.797077087897755,0.794518382245735,
9.16992696032854));
#10636=CARTESIAN_POINT('Ctrl Pts',(-1.09856425898481,0.249118120983399,
9.19900933156918));
#10637=CARTESIAN_POINT('Ctrl Pts',(-1.06380000922336,-0.374144935055997,
9.22811991749506));
#10638=CARTESIAN_POINT('Ctrl Pts',(-0.769172046065886,-0.788482110834251,
9.25185920107736));
#10639=CARTESIAN_POINT('Ctrl Pts',(-0.367182194896042,-1.03416770199381,
9.27453758860991));
#10640=CARTESIAN_POINT('Ctrl Pts',(0.0395215134476794,-1.10612289271203,
9.29398716301566));
#10641=CARTESIAN_POINT('Ctrl Pts',(0.477622137462348,-0.988239329641883,
9.315608935922));
#10642=CARTESIAN_POINT('Ctrl Pts',(0.806060476953854,-0.746133466732723,
9.33508059295667));
#10643=CARTESIAN_POINT('Ctrl Pts',(1.02338097622177,-0.400209794823969,
9.35455900998878));
#10644=CARTESIAN_POINT('Ctrl Pts',(1.09301857284269,-0.0322005400116846,
9.37242337753565));
#10645=CARTESIAN_POINT('Ctrl Pts',(1.04557123688016,0.302448473621783,9.38867049786501));
#10646=CARTESIAN_POINT('Ctrl Pts',(0.880248597472728,0.673138628508302,
9.40817382201824));
#10647=CARTESIAN_POINT('Ctrl Pts',(0.490987821358575,1.0215162740493,9.43255931556892));
#10648=CARTESIAN_POINT('Ctrl Pts',(-0.128028731061003,1.12673431002624,
9.46184150098951));
#10649=CARTESIAN_POINT('Ctrl Pts',(-0.611115346897492,0.92634451080831,
9.48625316647187));
#10650=CARTESIAN_POINT('Ctrl Pts',(-0.890003906782786,0.630491031563606,
9.50579262818851));
#10651=CARTESIAN_POINT('Ctrl Pts',(-1.07718613810329,0.269493001893084,
9.52533614230101));
#10652=CARTESIAN_POINT('Ctrl Pts',(-1.10685316099274,-0.253206849806021,
9.549769143617));
#10653=CARTESIAN_POINT('Ctrl Pts',(-0.802665388553327,-0.80350029659764,
9.57910079014067));
#10654=CARTESIAN_POINT('Ctrl Pts',(-0.252382142420839,-1.10765434668513,
9.60844033627772));
#10655=CARTESIAN_POINT('Ctrl Pts',(0.375622844421776,-1.07241880015879,
9.6377872616149));
#10656=CARTESIAN_POINT('Ctrl Pts',(0.888675653575918,-0.708384464521095,
9.66713948562636));
#10657=CARTESIAN_POINT('Ctrl Pts',(1.12945283978432,-0.127110607216331,
9.69649562191789));
#10658=CARTESIAN_POINT('Ctrl Pts',(1.02406436855865,0.493221535835591,9.72585399659149));
#10659=CARTESIAN_POINT('Ctrl Pts',(0.604750564115747,0.962410167163729,
9.75521300373452));
#10660=CARTESIAN_POINT('Ctrl Pts',(0.00018168777481138,1.13659797379318,
9.78457113260792));
#10661=CARTESIAN_POINT('Ctrl Pts',(-0.604514012247553,0.962442862813792,
9.81392653168396));
#10662=CARTESIAN_POINT('Ctrl Pts',(-1.00788755091294,0.510743356018493,
9.84219098822073));
#10663=CARTESIAN_POINT('Ctrl Pts',(-1.12223084029966,-0.0555269185822364,
9.86936284287987));
#10664=CARTESIAN_POINT('Ctrl Pts',(-0.958681149169006,-0.584986935290896,
9.89544464218138));
#10665=CARTESIAN_POINT('Ctrl Pts',(-0.595072606804766,-0.939890399434298,
9.91934680514532));
#10666=CARTESIAN_POINT('Ctrl Pts',(-0.165261742340907,-1.08943840079317,
9.94106900696797));
#10667=CARTESIAN_POINT('Ctrl Pts',(0.381501891532602,-1.07053143388919,
9.96713134343117));
#10668=CARTESIAN_POINT('Ctrl Pts',(0.856595948124104,-0.748119235797807,
9.99318006438684));
#10669=CARTESIAN_POINT('Ctrl Pts',(1.07309034940253,-0.246007820424173,
10.0192184485331));
#10670=CARTESIAN_POINT('Ctrl Pts',(1.09532486422704,0.299243704641549,10.0452489336159));
#10671=CARTESIAN_POINT('Ctrl Pts',(0.737208771049273,0.921717292357175,
10.0777646557385));
#10672=CARTESIAN_POINT('Ctrl Pts',(-0.0875976639157576,1.17590238091633,
10.1167545687155));
#10673=CARTESIAN_POINT('Ctrl Pts',(-0.775414432101575,0.843148981901611,
10.1513791941553));
#10674=CARTESIAN_POINT('Ctrl Pts',(-1.08237439891738,0.276792097832271,
10.1816522621836));
#10675=CARTESIAN_POINT('Ctrl Pts',(-1.08223987573992,-0.273905699897673,
10.2075837109931));
#10676=CARTESIAN_POINT('Ctrl Pts',(-0.819021356744807,-0.757885892152692,
10.2334953587529));
#10677=CARTESIAN_POINT('Ctrl Pts',(-0.35659410762715,-1.05617411390235,
10.2593858505813));
#10678=CARTESIAN_POINT('Ctrl Pts',(0.191709377129806,-1.09707930859612,
10.2852567627067));
#10679=CARTESIAN_POINT('Ctrl Pts',(0.619305370577929,-0.903938602256031,
10.307333480538));
#10680=CARTESIAN_POINT('Ctrl Pts',(0.880476818061234,-0.627047684176173,
10.3256298718571));
#10681=CARTESIAN_POINT('Ctrl Pts',(1.0658885916031,-0.26934857845919,10.3449924871254));
#10682=CARTESIAN_POINT('Ctrl Pts',(1.09515715586536,0.247897726642305,10.3691745552382));
#10683=CARTESIAN_POINT('Ctrl Pts',(0.794434828137204,0.79164810257108,10.3981621507212));
#10684=CARTESIAN_POINT('Ctrl Pts',(0.2513627005957,1.09165703572537,10.4271160993126));
#10685=CARTESIAN_POINT('Ctrl Pts',(-0.367454430252698,1.05680897175568,
10.4560357085573));
#10686=CARTESIAN_POINT('Ctrl Pts',(-0.872209226186921,0.698502678542679,
10.4849194330614));
#10687=CARTESIAN_POINT('Ctrl Pts',(-1.10868326692617,0.127308218351685,
10.5137661629812));
#10688=CARTESIAN_POINT('Ctrl Pts',(-1.00514471501034,-0.48133956103109,
10.5425746368362));
#10689=CARTESIAN_POINT('Ctrl Pts',(-0.594223537283247,-0.940976300734034,
10.5713437045289));
#10690=CARTESIAN_POINT('Ctrl Pts',(-0.002580678613507,-1.11129495562103,
10.6000722203793));
#10691=CARTESIAN_POINT('Ctrl Pts',(0.588129815347979,-0.940979629269841,
10.6287590718095));
#10692=CARTESIAN_POINT('Ctrl Pts',(0.997070643975556,-0.483175565710426,
10.6574031830034));
#10693=CARTESIAN_POINT('Ctrl Pts',(1.09960229356506,0.121100802476138,10.6860035048011));
#10694=CARTESIAN_POINT('Ctrl Pts',(0.86528778983678,0.686415227285098,10.7145590265277));
#10695=CARTESIAN_POINT('Ctrl Pts',(0.366920420197264,1.03984587815201,10.7430687635858));
#10696=CARTESIAN_POINT('Ctrl Pts',(-0.242097189914162,1.0738946711142,10.7715317681828));
#10697=CARTESIAN_POINT('Ctrl Pts',(-0.774990713253418,0.779200373976015,
10.7999471270303));
#10698=CARTESIAN_POINT('Ctrl Pts',(-1.06891817459263,0.2470593867986,10.8283139593686));
#10699=CARTESIAN_POINT('Ctrl Pts',(-1.03474665817,-0.358829623525622,10.8566314075575));
#10700=CARTESIAN_POINT('Ctrl Pts',(-0.684094896882393,-0.85283074565291,
10.8848986782965));
#10701=CARTESIAN_POINT('Ctrl Pts',(-0.125405267425638,-1.0840777799931,
10.9131149316417));
#10702=CARTESIAN_POINT('Ctrl Pts',(0.469566204102857,-0.982999822886529,
10.9412795295327));
#10703=CARTESIAN_POINT('Ctrl Pts',(0.918640045850225,-0.581294038472193,
10.9693914839116));
#10704=CARTESIAN_POINT('Ctrl Pts',(1.02944056689496,-0.1965869628994,10.9880983243323));
#10705=CARTESIAN_POINT('Ctrl Pts',(1.02946655913226,-0.00351001149624692,
10.997442756416));
#10706=CARTESIAN_POINT('Ctrl Pts',(0.932816117174745,0.00257753706438406,
7.82155541886881));
#10707=CARTESIAN_POINT('Ctrl Pts',(0.932792537460822,0.177733635780523,
7.83003252737339));
#10708=CARTESIAN_POINT('Ctrl Pts',(0.832395790527212,0.526201721661573,
7.84697613681209));
#10709=CARTESIAN_POINT('Ctrl Pts',(0.425544200513314,0.890172337838447,
7.87244618255503));
#10710=CARTESIAN_POINT('Ctrl Pts',(-0.11336388666004,0.98167567131432,7.89795412018352));
#10711=CARTESIAN_POINT('Ctrl Pts',(-0.61933707944609,0.772243525278785,
7.92350765312756));
#10712=CARTESIAN_POINT('Ctrl Pts',(-0.936881339315919,0.324863039572081,
7.94910507894627));
#10713=CARTESIAN_POINT('Ctrl Pts',(-0.96782639358118,-0.223839618027314,
7.97474887367392));
#10714=CARTESIAN_POINT('Ctrl Pts',(-0.701621350606369,-0.705803746925262,
8.00043961028665));
#10715=CARTESIAN_POINT('Ctrl Pts',(-0.218907478333097,-0.972762223001147,
8.02617867435414));
#10716=CARTESIAN_POINT('Ctrl Pts',(0.332899340942218,-0.941930890565723,
8.0519670470666));
#10717=CARTESIAN_POINT('Ctrl Pts',(0.78460355937521,-0.62162490930732,8.07780583779769));
#10718=CARTESIAN_POINT('Ctrl Pts',(0.997079900383295,-0.109076731898229,
8.10369604591022));
#10719=CARTESIAN_POINT('Ctrl Pts',(0.904115937338599,0.439056301982027,
8.12963867407103));
#10720=CARTESIAN_POINT('Ctrl Pts',(0.533006028155458,0.854574243625169,
8.1556346512764));
#10721=CARTESIAN_POINT('Ctrl Pts',(-0.0033797306614811,1.00926211236485,
8.18168490546527));
#10722=CARTESIAN_POINT('Ctrl Pts',(-0.541040252974749,0.854578896037574,
8.2077902454942));
#10723=CARTESIAN_POINT('Ctrl Pts',(-0.900819615004692,0.452035261399126,
8.232982646847));
#10724=CARTESIAN_POINT('Ctrl Pts',(-0.986407683770965,0.0272443707704438,
8.25337195355103));
#10725=CARTESIAN_POINT('Ctrl Pts',(-0.937109814892794,-0.251094083734033,
8.26698515637403));
#10726=CARTESIAN_POINT('Ctrl Pts',(-0.880272398528943,-0.401369554301966,
8.27476997312653));
#10727=CARTESIAN_POINT('Ctrl Pts',(-0.767699859183187,-0.614677280654596,
8.28645287628459));
#10728=CARTESIAN_POINT('Ctrl Pts',(-0.50103538805602,-0.874994963856704,
8.30399768727805));
#10729=CARTESIAN_POINT('Ctrl Pts',(-0.0213267761989935,-1.01048232574384,
8.3274382097326));
#10730=CARTESIAN_POINT('Ctrl Pts',(0.464863835130203,-0.898942626339521,
8.35092523032543));
#10731=CARTESIAN_POINT('Ctrl Pts',(0.903709188564727,-0.513852403673233,
8.378381904535));
#10732=CARTESIAN_POINT('Ctrl Pts',(1.05988003651373,0.163448042572348,8.40983937592686));
#10733=CARTESIAN_POINT('Ctrl Pts',(0.710583436266589,0.766752724788841,
8.44139319618407));
#10734=CARTESIAN_POINT('Ctrl Pts',(0.1735498784337,1.0078575404005,8.46907468175037));
#10735=CARTESIAN_POINT('Ctrl Pts',(-0.329995702322566,0.970390012101335,
8.49285073236006));
#10736=CARTESIAN_POINT('Ctrl Pts',(-0.720223604553968,0.718362602848667,
8.51469007548597));
#10737=CARTESIAN_POINT('Ctrl Pts',(-0.941451908882603,0.365265796603737,
8.53458030754323));
#10738=CARTESIAN_POINT('Ctrl Pts',(-1.03626047645768,-0.127279523370467,
8.55848580751551));
#10739=CARTESIAN_POINT('Ctrl Pts',(-0.795928784219165,-0.74311800603862,
8.58843676936027));
#10740=CARTESIAN_POINT('Ctrl Pts',(-0.0776928783325622,-1.08960753239903,
8.62449067399998));
#10741=CARTESIAN_POINT('Ctrl Pts',(0.685958843373295,-0.854222896365132,
8.6606570762863));
#10742=CARTESIAN_POINT('Ctrl Pts',(1.08739997467006,-0.160417924516188,
8.6969363405203));
#10743=CARTESIAN_POINT('Ctrl Pts',(0.908689963674042,0.624433563761331,
8.73332847548848));
#10744=CARTESIAN_POINT('Ctrl Pts',(0.35355644738896,1.00221415934711,8.76374905337087));
#10745=CARTESIAN_POINT('Ctrl Pts',(-0.157958762417835,1.01991936283588,
8.788141995761));
#10746=CARTESIAN_POINT('Ctrl Pts',(-0.560829075860804,0.87964148645711,
8.80850060768873));
#10747=CARTESIAN_POINT('Ctrl Pts',(-0.902376151855375,0.546783264171767,
8.83093497234893));
#10748=CARTESIAN_POINT('Ctrl Pts',(-1.05620262261865,0.0487131824532962,
8.85545846822155));
#10749=CARTESIAN_POINT('Ctrl Pts',(-0.952659486533578,-0.46308305095605,
8.88003143979645));
#10750=CARTESIAN_POINT('Ctrl Pts',(-0.616438751614575,-0.864172093596548,
8.90465367965298));
#10751=CARTESIAN_POINT('Ctrl Pts',(-0.128491501662308,-1.05563283300167,
8.929324858834));
#10752=CARTESIAN_POINT('Ctrl Pts',(0.349568464277159,-0.995857144249034,
8.95198485171474));
#10753=CARTESIAN_POINT('Ctrl Pts',(0.715092597634469,-0.765243557764514,
8.97262009973951));
#10754=CARTESIAN_POINT('Ctrl Pts',(1.02585817273875,-0.347854923658281,
8.99741854820384));
#10755=CARTESIAN_POINT('Ctrl Pts',(1.07902066886242,0.335854720189213,9.02848390246269));
#10756=CARTESIAN_POINT('Ctrl Pts',(0.64850518863454,0.874001973235243,9.05963864033205));
#10757=CARTESIAN_POINT('Ctrl Pts',(0.153754709377709,1.04541750824584,9.08461452336056));
#10758=CARTESIAN_POINT('Ctrl Pts',(-0.304660404754024,1.02923830963297,
9.10649891467337));
#10759=CARTESIAN_POINT('Ctrl Pts',(-0.774772226567215,0.769734721067703,
9.13155302818068));
#10760=CARTESIAN_POINT('Ctrl Pts',(-1.06758176764164,0.240194096660453,
9.15979645527093));
#10761=CARTESIAN_POINT('Ctrl Pts',(-1.03388209497993,-0.365632688574458,
9.1880966422963));
#10762=CARTESIAN_POINT('Ctrl Pts',(-0.747236634374738,-0.768864123830532,
9.21120196811848));
#10763=CARTESIAN_POINT('Ctrl Pts',(-0.355793348154831,-1.0081210605673,
9.23328752841953));
#10764=CARTESIAN_POINT('Ctrl Pts',(0.0405271187519368,-1.0782861333172,
9.25224234259836));
#10765=CARTESIAN_POINT('Ctrl Pts',(0.467851885055523,-0.963334110221332,
9.27333469283053));
#10766=CARTESIAN_POINT('Ctrl Pts',(0.788437476668796,-0.727044639163456,
9.2923412041483));
#10767=CARTESIAN_POINT('Ctrl Pts',(1.0007528826234,-0.389147467838417,9.3113715890792));
#10768=CARTESIAN_POINT('Ctrl Pts',(1.06885322196228,-0.0293996181272015,
9.32883720111315));
#10769=CARTESIAN_POINT('Ctrl Pts',(1.02245490094734,0.297953905849491,9.34473160287988));
#10770=CARTESIAN_POINT('Ctrl Pts',(0.86066371709643,0.660768124405153,9.36382175120697));
#10771=CARTESIAN_POINT('Ctrl Pts',(0.479374090360282,1.00212138313223,9.38771687527452));
#10772=CARTESIAN_POINT('Ctrl Pts',(-0.127718095046861,1.10542227002233,
9.41643972739237));
#10773=CARTESIAN_POINT('Ctrl Pts',(-0.602123430277001,0.90873622757722,
9.4404161706225));
#10774=CARTESIAN_POINT('Ctrl Pts',(-0.876217908012786,0.617994917673252,
9.45962012033667));
#10775=CARTESIAN_POINT('Ctrl Pts',(-1.06029538877664,0.263022921439863,
9.47883959441989));
#10776=CARTESIAN_POINT('Ctrl Pts',(-1.08958045724843,-0.25145714410997,
9.50289353969035));
#10777=CARTESIAN_POINT('Ctrl Pts',(-0.789910095070733,-0.793793425585321,
9.53180255933616));
#10778=CARTESIAN_POINT('Ctrl Pts',(-0.247026510336,-1.09398288546205,9.56075524452346));
#10779=CARTESIAN_POINT('Ctrl Pts',(0.373354429623973,-1.05928378029671,
9.58975007442778));
#10780=CARTESIAN_POINT('Ctrl Pts',(0.880858555852544,-0.699321360637946,
9.61878586997401));
#10781=CARTESIAN_POINT('Ctrl Pts',(1.11939651791946,-0.123739308088276,
9.64786125750938));
#10782=CARTESIAN_POINT('Ctrl Pts',(1.01501061604786,0.491341759208262,9.67697489434579));
#10783=CARTESIAN_POINT('Ctrl Pts',(0.598822393739831,0.957195198398869,
9.70612540386286));
#10784=CARTESIAN_POINT('Ctrl Pts',(-0.00207634075492403,1.13043680813235,
9.73531134564448));
#10785=CARTESIAN_POINT('Ctrl Pts',(-0.603912123248523,0.957215276033718,
9.76453137942698));
#10786=CARTESIAN_POINT('Ctrl Pts',(-1.00594389361736,0.507177516237079,
9.79270042150575));
#10787=CARTESIAN_POINT('Ctrl Pts',(-1.12009446569155,-0.0577553123758345,
9.81981342467293));
#10788=CARTESIAN_POINT('Ctrl Pts',(-0.956831265840032,-0.586568536389845,
9.8458643888034));
#10789=CARTESIAN_POINT('Ctrl Pts',(-0.593322824365002,-0.941465991223857,
9.8697649885894));
#10790=CARTESIAN_POINT('Ctrl Pts',(-0.163152777889603,-1.09117482218559,
9.89150891502364));
#10791=CARTESIAN_POINT('Ctrl Pts',(0.384507054175381,-1.07229194200837,
9.91761601463539));
#10792=CARTESIAN_POINT('Ctrl Pts',(0.861095137732964,-0.749070261446909,
9.94374661664145));
#10793=CARTESIAN_POINT('Ctrl Pts',(1.07855069686503,-0.24487939037421,9.96989644300623));
#10794=CARTESIAN_POINT('Ctrl Pts',(1.10093949076505,0.303072931485129,9.9960586104448));
#10795=CARTESIAN_POINT('Ctrl Pts',(0.74077341907722,0.929563584544601,10.0287865624482));
#10796=CARTESIAN_POINT('Ctrl Pts',(-0.0904825710551195,1.18602420370029,
10.0680912360091));
#10797=CARTESIAN_POINT('Ctrl Pts',(-0.785003918826264,0.850284549087302,
10.1030550955328));
#10798=CARTESIAN_POINT('Ctrl Pts',(-1.0954014372141,0.277765624320416,10.1336635590215));
#10799=CARTESIAN_POINT('Ctrl Pts',(-1.09534339945125,-0.279543559457623,
10.1599082341136));
#10800=CARTESIAN_POINT('Ctrl Pts',(-0.828733022228398,-0.769900103510982,
10.1861618892393));
#10801=CARTESIAN_POINT('Ctrl Pts',(-0.359774220131184,-1.07248984309679,
10.212423484559));
#10802=CARTESIAN_POINT('Ctrl Pts',(0.196885914186667,-1.11409518777613,
10.2386900633088));
#10803=CARTESIAN_POINT('Ctrl Pts',(0.631515451668511,-0.917851149722072,
10.2611320934233));
#10804=CARTESIAN_POINT('Ctrl Pts',(0.897179887249006,-0.636222443941654,
10.2797433547922));
#10805=CARTESIAN_POINT('Ctrl Pts',(1.0858961146808,-0.272190094723938,10.2994507035648));
#10806=CARTESIAN_POINT('Ctrl Pts',(1.11580087037807,0.254712868751099,10.3240884429413));
#10807=CARTESIAN_POINT('Ctrl Pts',(0.809208599810454,0.809296967356682,
10.353654139103));
#10808=CARTESIAN_POINT('Ctrl Pts',(0.254788423957568,1.11569881651034,10.383219698794));
#10809=CARTESIAN_POINT('Ctrl Pts',(-0.377734849108055,1.08018316957416,
10.4127829355374));
#10810=CARTESIAN_POINT('Ctrl Pts',(-0.894297933370396,0.713620441102003,
10.4423423586806));
#10811=CARTESIAN_POINT('Ctrl Pts',(-1.13663484410025,0.128525956779319,
10.4718961659386));
#10812=CARTESIAN_POINT('Ctrl Pts',(-1.03055159767899,-0.495666761823774,
10.5014426885714));
#10813=CARTESIAN_POINT('Ctrl Pts',(-0.608768055200784,-0.967598798699277,
10.5309801966361));
#10814=CARTESIAN_POINT('Ctrl Pts',(-0.000768715985731294,-1.14272525987886,
10.5605070077873));
#10815=CARTESIAN_POINT('Ctrl Pts',(0.606953484275095,-0.967602860308774,
10.5900214114748));
#10816=CARTESIAN_POINT('Ctrl Pts',(1.02815040642715,-0.496217147831501,
10.6195217311575));
#10817=CARTESIAN_POINT('Ctrl Pts',(1.13393293838566,0.126674177284328,10.6490062827704));
#10818=CARTESIAN_POINT('Ctrl Pts',(0.892240327216091,0.710023030082336,
10.6784734108048));
#10819=CARTESIAN_POINT('Ctrl Pts',(0.37756151121538,1.0751290249391,10.7079214511558));
#10820=CARTESIAN_POINT('Ctrl Pts',(-0.252037482971,1.11041475463464,10.7373487814911));
#10821=CARTESIAN_POINT('Ctrl Pts',(-0.803490717852888,0.805552343975863,
10.7667537501932));
#10822=CARTESIAN_POINT('Ctrl Pts',(-1.10797664005012,0.254464265888738,
10.796134828178));
#10823=CARTESIAN_POINT('Ctrl Pts',(-1.07263280292657,-0.373598325782701,
10.8254902498732));
#10824=CARTESIAN_POINT('Ctrl Pts',(-0.708901590711751,-0.88615095694047,
10.8548188612348));
#10825=CARTESIAN_POINT('Ctrl Pts',(-0.128820897427331,-1.12633619172926,
10.8841182058041));
#10826=CARTESIAN_POINT('Ctrl Pts',(0.489474256939415,-1.02135047902734,
10.9133888202114));
#10827=CARTESIAN_POINT('Ctrl Pts',(0.956556872453774,-0.603666350937339,
10.9426246469134));
#10828=CARTESIAN_POINT('Ctrl Pts',(1.07193781572403,-0.203201562396062,
10.9621000587781));
#10829=CARTESIAN_POINT('Ctrl Pts',(1.07196486456811,-0.00227586712733216,
10.9718243500499));
#10830=CARTESIAN_POINT('Ctrl Pts',(0.916386464361943,-0.00093309831050743,
7.8940473292219));
#10831=CARTESIAN_POINT('Ctrl Pts',(0.916363306673161,0.171088090561208,
7.90237271608449));
#10832=CARTESIAN_POINT('Ctrl Pts',(0.817709848796121,0.513018539755372,
7.91900290782367));
#10833=CARTESIAN_POINT('Ctrl Pts',(0.419193318564387,0.869300720967443,
7.94394562555401));
#10834=CARTESIAN_POINT('Ctrl Pts',(-0.107459845420563,0.958570197177955,
7.96887498479583));
#10835=CARTESIAN_POINT('Ctrl Pts',(-0.600815190480234,0.754199282249767,
7.99379660366029));
#10836=CARTESIAN_POINT('Ctrl Pts',(-0.90972475540008,0.318735876207034,
8.01871040893382));
#10837=CARTESIAN_POINT('Ctrl Pts',(-0.939634168320183,-0.214178713135979,
8.04361889595454));
#10838=CARTESIAN_POINT('Ctrl Pts',(-0.681480351317133,-0.681266235779645,
8.06852342334305));
#10839=CARTESIAN_POINT('Ctrl Pts',(-0.214442030770815,-0.939390273067314,
8.0934258663209));
#10840=CARTESIAN_POINT('Ctrl Pts',(0.318328618727776,-0.909478985290061,
8.11832788264496));
#10841=CARTESIAN_POINT('Ctrl Pts',(0.753548017202942,-0.600689198431121,
8.14323122154075));
#10842=CARTESIAN_POINT('Ctrl Pts',(0.957798608325141,-0.107620541089113,
8.16813759793459));
#10843=CARTESIAN_POINT('Ctrl Pts',(0.868405979460084,0.418636976277688,
8.19304874272053));
#10844=CARTESIAN_POINT('Ctrl Pts',(0.512629065363514,0.816784590937834,
8.21796638811051));
#10845=CARTESIAN_POINT('Ctrl Pts',(-0.000585672768811046,0.964652867330779,
8.24289223431723));
#10846=CARTESIAN_POINT('Ctrl Pts',(-0.514067682434154,0.816790328676347,
8.26782807268141));
#10847=CARTESIAN_POINT('Ctrl Pts',(-0.857028397869778,0.432886852605677,
8.29185151518157));
#10848=CARTESIAN_POINT('Ctrl Pts',(-0.938441693019448,0.0284593721668554,
8.31126498760023));
#10849=CARTESIAN_POINT('Ctrl Pts',(-0.891549619244174,-0.236233682506208,
8.32421168378805));
#10850=CARTESIAN_POINT('Ctrl Pts',(-0.837526115658479,-0.379066140937872,
8.33161111168448));
#10851=CARTESIAN_POINT('Ctrl Pts',(-0.730561974805884,-0.581738446354059,
8.34271189331387));
#10852=CARTESIAN_POINT('Ctrl Pts',(-0.477352425520727,-0.828842529403336,
8.35937075304238));
#10853=CARTESIAN_POINT('Ctrl Pts',(-0.0225330382004105,-0.957209024892203,
8.38159488569873));
#10854=CARTESIAN_POINT('Ctrl Pts',(0.437788178382466,-0.851537961861344,
8.40383465770076));
#10855=CARTESIAN_POINT('Ctrl Pts',(0.852715694662685,-0.487307649407337,
8.42980009152249));
#10856=CARTESIAN_POINT('Ctrl Pts',(0.999965381191419,0.152241057725198,
8.45950561391401));
#10857=CARTESIAN_POINT('Ctrl Pts',(0.670567292988393,0.720763590006567,
8.48924952521388));
#10858=CARTESIAN_POINT('Ctrl Pts',(0.165104121582195,0.947610229347272,
8.51530399445417));
#10859=CARTESIAN_POINT('Ctrl Pts',(-0.308304372080754,0.912327630374344,
8.53765800829594));
#10860=CARTESIAN_POINT('Ctrl Pts',(-0.67477683344297,0.675573610699686,
8.55817118909699));
#10861=CARTESIAN_POINT('Ctrl Pts',(-0.882350277706418,0.34422728689363,
8.57683651179162));
#10862=CARTESIAN_POINT('Ctrl Pts',(-0.971219773321951,-0.117642462843675,
8.59925338393781));
#10863=CARTESIAN_POINT('Ctrl Pts',(-0.745953604143611,-0.694472541682851,
8.62731233232217));
#10864=CARTESIAN_POINT('Ctrl Pts',(-0.0739633240472909,-1.01845581262107,
8.66104313406658));
#10865=CARTESIAN_POINT('Ctrl Pts',(0.63952747451705,-0.798369631564053,
8.69483872901917));
#10866=CARTESIAN_POINT('Ctrl Pts',(1.01408422655149,-0.150734124008621,
8.72870212818689));
#10867=CARTESIAN_POINT('Ctrl Pts',(0.847322126498796,0.58103611525318,8.76263640124927));
#10868=CARTESIAN_POINT('Ctrl Pts',(0.330121026915543,0.932886604391724,
8.79097752783638));
#10869=CARTESIAN_POINT('Ctrl Pts',(-0.146093769553075,0.949351984337242,
8.81368784917009));
#10870=CARTESIAN_POINT('Ctrl Pts',(-0.521021746649022,0.818789575072917,
8.83263515205418));
#10871=CARTESIAN_POINT('Ctrl Pts',(-0.838737700087821,0.509122269324307,
8.85350597952678));
#10872=CARTESIAN_POINT('Ctrl Pts',(-0.981754612397829,0.0459670008233027,
8.87631102562348));
#10873=CARTESIAN_POINT('Ctrl Pts',(-0.885491145123779,-0.429752885191932,
8.89915236426619));
#10874=CARTESIAN_POINT('Ctrl Pts',(-0.573052273480284,-0.802442728830194,
8.9220328462699));
#10875=CARTESIAN_POINT('Ctrl Pts',(-0.11977334499688,-0.980285495206635,
8.94495124212259));
#10876=CARTESIAN_POINT('Ctrl Pts',(0.324211584585207,-0.924759915662738,
8.96599677624005));
#10877=CARTESIAN_POINT('Ctrl Pts',(0.663619579763974,-0.710620166507527,
8.98515810751412));
#10878=CARTESIAN_POINT('Ctrl Pts',(0.952143685172452,-0.323095904167005,
9.00818238284112));
#10879=CARTESIAN_POINT('Ctrl Pts',(1.00147844946261,0.311593665089388,9.03702060642391));
#10880=CARTESIAN_POINT('Ctrl Pts',(0.601866958953658,0.811110161437164,
9.06593988482292));
#10881=CARTESIAN_POINT('Ctrl Pts',(0.142635782304362,0.970222188044987,
9.08912285438075));
#10882=CARTESIAN_POINT('Ctrl Pts',(-0.282880216341775,0.955206494432585,
9.10943681406231));
#10883=CARTESIAN_POINT('Ctrl Pts',(-0.719285418358596,0.714319703027661,
9.13269449197724));
#10884=CARTESIAN_POINT('Ctrl Pts',(-0.991145548172263,0.222695996518761,
9.1589160433785));
#10885=CARTESIAN_POINT('Ctrl Pts',(-0.9598723234409,-0.33986314694992,9.18519504623541));
#10886=CARTESIAN_POINT('Ctrl Pts',(-0.693651734536496,-0.714395587302459,
9.20665515597952));
#10887=CARTESIAN_POINT('Ctrl Pts',(-0.33000558647281,-0.936668388183705,
9.22717248577931));
#10888=CARTESIAN_POINT('Ctrl Pts',(0.0382488951801815,-1.00187881354344,
9.24478504858718));
#10889=CARTESIAN_POINT('Ctrl Pts',(0.435428514213863,-0.895048693578503,
9.26438909498248));
#10890=CARTESIAN_POINT('Ctrl Pts',(0.733481601998805,-0.67537933957951,
9.28205927527633));
#10891=CARTESIAN_POINT('Ctrl Pts',(0.930935942815539,-0.361155740600938,
9.29975646442145));
#10892=CARTESIAN_POINT('Ctrl Pts',(0.994297368624369,-0.0265033935802915,
9.31600357587152));
#10893=CARTESIAN_POINT('Ctrl Pts',(0.951128789628544,0.278106881586742,
9.33079344806764));
#10894=CARTESIAN_POINT('Ctrl Pts',(0.800547029468414,0.615803482990443,
9.34856170352529));
#10895=CARTESIAN_POINT('Ctrl Pts',(0.445541906176031,0.933679329429137,
9.37081057426095));
#10896=CARTESIAN_POINT('Ctrl Pts',(-0.120075741503171,1.02997680518912,
9.39757104683856));
#10897=CARTESIAN_POINT('Ctrl Pts',(-0.562380172430049,0.846648767025865,
9.41992332291532));
#10898=CARTESIAN_POINT('Ctrl Pts',(-0.818063047449599,0.575452122500431,
9.43783641698758));
#10899=CARTESIAN_POINT('Ctrl Pts',(-0.989839448666035,0.24422322307351,
9.45577041101522));
#10900=CARTESIAN_POINT('Ctrl Pts',(-1.01723457777004,-0.236110259423285,
9.47822706382322));
#10901=CARTESIAN_POINT('Ctrl Pts',(-0.737289662342792,-0.742891434307192,
9.50523810407958));
#10902=CARTESIAN_POINT('Ctrl Pts',(-0.229642005372076,-1.02367828901602,
9.53231229849314));
#10903=CARTESIAN_POINT('Ctrl Pts',(0.351027390123253,-0.991276097967053,
9.559449788874));
#10904=CARTESIAN_POINT('Ctrl Pts',(0.826527285725571,-0.654110782122341,
9.58665063199169));
#10905=CARTESIAN_POINT('Ctrl Pts',(1.05029403858789,-0.11438813617086,9.61391485224451));
#10906=CARTESIAN_POINT('Ctrl Pts',(0.952393012397771,0.463003902808121,
9.64124242605231));
#10907=CARTESIAN_POINT('Ctrl Pts',(0.561373841868419,0.900822151844062,
9.66863326977439));
#10908=CARTESIAN_POINT('Ctrl Pts',(-0.00387276695331408,1.0638843291464,
9.69608728519562));
#10909=CARTESIAN_POINT('Ctrl Pts',(-0.570695551262971,0.900845596732101,
9.723604249157));
#10910=CARTESIAN_POINT('Ctrl Pts',(-0.949833801943534,0.476579569449792,
9.75016258055998));
#10911=CARTESIAN_POINT('Ctrl Pts',(-1.05766462295084,-0.0566720978017236,
9.77575398707171));
#10912=CARTESIAN_POINT('Ctrl Pts',(-0.903446650287503,-0.556425680500337,
9.80037141569279));
#10913=CARTESIAN_POINT('Ctrl Pts',(-0.55959314493252,-0.892235666458625,
9.82298223779303));
#10914=CARTESIAN_POINT('Ctrl Pts',(-0.152220323052832,-1.03404623235443,
9.84357273851314));
#10915=CARTESIAN_POINT('Ctrl Pts',(0.366883172029728,-1.01619539695405,
9.86831820213365));
#10916=CARTESIAN_POINT('Ctrl Pts',(0.819317002651662,-0.709565750262104,
9.89311712889566));
#10917=CARTESIAN_POINT('Ctrl Pts',(1.02605541148877,-0.230354394394416,
9.91797028804756));
#10918=CARTESIAN_POINT('Ctrl Pts',(1.04740076386437,0.290941337297571,9.94285927862722));
#10919=CARTESIAN_POINT('Ctrl Pts',(0.704487085949529,0.887918159178826,
9.97403534857104));
#10920=CARTESIAN_POINT('Ctrl Pts',(-0.0889329641953167,1.13305086915798,
10.0115520936496));
#10921=CARTESIAN_POINT('Ctrl Pts',(-0.753378607817973,0.812154603631431,
10.0449913261173));
#10922=CARTESIAN_POINT('Ctrl Pts',(-1.0509061430146,0.2636345725963,10.0743168693977));
#10923=CARTESIAN_POINT('Ctrl Pts',(-1.05093739784869,-0.271120657455177,
10.0994981767143));
#10924=CARTESIAN_POINT('Ctrl Pts',(-0.794853058550813,-0.742337793921308,
10.1247231042996));
#10925=CARTESIAN_POINT('Ctrl Pts',(-0.343652569312813,-1.03358848122898,
10.1499909616499));
#10926=CARTESIAN_POINT('Ctrl Pts',(0.192775959815744,-1.07377917166597,
10.1753023818525));
#10927=CARTESIAN_POINT('Ctrl Pts',(0.612246298230531,-0.884472212478353,
10.1969571970733));
#10928=CARTESIAN_POINT('Ctrl Pts',(0.868951664888123,-0.612372118526421,
10.2149387020014));
#10929=CARTESIAN_POINT('Ctrl Pts',(1.05146362716697,-0.260359176846704,
10.2339952372064));
#10930=CARTESIAN_POINT('Ctrl Pts',(1.08053751648403,0.249785530435256,10.2578467531362));
#10931=CARTESIAN_POINT('Ctrl Pts',(0.783308174548958,0.787746446449566,
10.2865196367573));
#10932=CARTESIAN_POINT('Ctrl Pts',(0.244719009240793,1.08556755291199,10.3152415913622));
#10933=CARTESIAN_POINT('Ctrl Pts',(-0.370909273962754,1.05115342677162,
10.3440118820671));
#10934=CARTESIAN_POINT('Ctrl Pts',(-0.874646110508742,0.693881654635859,
10.3728291813908));
#10935=CARTESIAN_POINT('Ctrl Pts',(-1.11148911187944,0.122460707441426,
10.4016923877211));
#10936=CARTESIAN_POINT('Ctrl Pts',(-1.00784436408095,-0.488329418075964,
10.4306002515908));
#10937=CARTESIAN_POINT('Ctrl Pts',(-0.594508503032201,-0.95104895241576,
10.4595515415207));
#10938=CARTESIAN_POINT('Ctrl Pts',(0.00252468810929164,-1.12318404866533,
10.4885449844876));
#10939=CARTESIAN_POINT('Ctrl Pts',(0.600466974195298,-0.951048000094383,
10.517579269984));
#10940=CARTESIAN_POINT('Ctrl Pts',(1.0157379397141,-0.486537895502348,10.5466530692494));
#10941=CARTESIAN_POINT('Ctrl Pts',(1.12035505762534,0.128518294750485,10.5757650148325));
#10942=CARTESIAN_POINT('Ctrl Pts',(0.881400098068042,0.705686601319807,
10.6049137245664));
#10943=CARTESIAN_POINT('Ctrl Pts',(0.371376215689227,1.06769185969133,10.6340977709503));
#10944=CARTESIAN_POINT('Ctrl Pts',(-0.253801011916156,1.10289557553796,
10.66331572853));
#10945=CARTESIAN_POINT('Ctrl Pts',(-0.802494827547404,0.799749660182247,
10.6925660997033));
#10946=CARTESIAN_POINT('Ctrl Pts',(-1.1061282469781,0.250555575979397,10.7218474788459));
#10947=CARTESIAN_POINT('Ctrl Pts',(-1.07100530702942,-0.376623977361633,
10.7511581664581));
#10948=CARTESIAN_POINT('Ctrl Pts',(-0.707253391080627,-0.88950243387736,
10.7804970768219));
#10949=CARTESIAN_POINT('Ctrl Pts',(-0.125893311798114,-1.13040111480947,
10.8098616956024));
#10950=CARTESIAN_POINT('Ctrl Pts',(0.495010447492726,-1.02512577517357,
10.8392526661857));
#10951=CARTESIAN_POINT('Ctrl Pts',(0.96503436836903,-0.605029576661258,
10.8686635500669));
#10952=CARTESIAN_POINT('Ctrl Pts',(1.08139545050083,-0.201364018273147,
10.8882928173859));
#10953=CARTESIAN_POINT('Ctrl Pts',(1.08142273213372,0.00129089154989864,
10.8981007982325));
#10954=CARTESIAN_POINT('Ctrl Pts',(0.962718053183473,-0.00374989906965716,
7.95237763337882));
#10955=CARTESIAN_POINT('Ctrl Pts',(0.962693741742924,0.176841650701835,
7.96111780385329));
#10956=CARTESIAN_POINT('Ctrl Pts',(0.859087970836183,0.535837040265186,
7.97857651794297));
#10957=CARTESIAN_POINT('Ctrl Pts',(0.44139204471531,0.909067672566069,8.00471126618545));
#10958=CARTESIAN_POINT('Ctrl Pts',(-0.10957037240375,1.00234938185105,8.03078957638873));
#10959=CARTESIAN_POINT('Ctrl Pts',(-0.624736766215092,0.788788067770214,
8.05681339506897));
#10960=CARTESIAN_POINT('Ctrl Pts',(-0.946645438372464,0.334753964295622,
8.08278312833397));
#10961=CARTESIAN_POINT('Ctrl Pts',(-0.977622131806228,-0.219795110452919,
8.10869993425576));
#10962=CARTESIAN_POINT('Ctrl Pts',(-0.709358577384567,-0.704866328363871,
8.1345646888734));
#10963=CARTESIAN_POINT('Ctrl Pts',(-0.225106799315938,-0.972333316118095,
8.16037844801135));
#10964=CARTESIAN_POINT('Ctrl Pts',(0.326150581648902,-0.94123300043997,
8.18614224392964));
#10965=CARTESIAN_POINT('Ctrl Pts',(0.775513506064428,-0.622221923030926,
8.21185716800189));
#10966=CARTESIAN_POINT('Ctrl Pts',(0.98588437082731,-0.113978011641057,
8.23752433345641));
#10967=CARTESIAN_POINT('Ctrl Pts',(0.893783701493479,0.427300464910859,
8.26314490422908));
#10968=CARTESIAN_POINT('Ctrl Pts',(0.528462068175506,0.835896897170472,
8.2887200485398));
#10969=CARTESIAN_POINT('Ctrl Pts',(0.00268624907551326,0.987222480008646,
8.31425101187734));
#10970=CARTESIAN_POINT('Ctrl Pts',(-0.522182866084098,0.835917649550696,
8.33973897090827));
#10971=CARTESIAN_POINT('Ctrl Pts',(-0.87192408794217,0.444190331151998,
8.36424287105709));
#10972=CARTESIAN_POINT('Ctrl Pts',(-0.954708318592613,0.0324397670437707,
8.3840047340831));
#10973=CARTESIAN_POINT('Ctrl Pts',(-0.9070179840126,-0.236658638349185,
8.39716640171874));
#10974=CARTESIAN_POINT('Ctrl Pts',(-0.852130113915824,-0.38176994593457,
8.40468374381179));
#10975=CARTESIAN_POINT('Ctrl Pts',(-0.74350765580059,-0.587578812177685,
8.41595591900598));
#10976=CARTESIAN_POINT('Ctrl Pts',(-0.486647878371642,-0.838127844696909,
8.43284869457147));
#10977=CARTESIAN_POINT('Ctrl Pts',(-0.0261984492433358,-0.967968322662697,
8.45534493147975));
#10978=CARTESIAN_POINT('Ctrl Pts',(0.438852361093423,-0.861090302172016,
8.47781287489012));
#10979=CARTESIAN_POINT('Ctrl Pts',(0.857189010370208,-0.493690220081531,
8.50399399075845));
#10980=CARTESIAN_POINT('Ctrl Pts',(1.00495380425253,0.149738205456235,8.53387052514169));
#10981=CARTESIAN_POINT('Ctrl Pts',(0.67426857107042,0.719767262233913,8.56369821016954));
#10982=CARTESIAN_POINT('Ctrl Pts',(0.168456706986281,0.946614776845862,
8.58976630720376));
#10983=CARTESIAN_POINT('Ctrl Pts',(-0.304308025339452,0.91126669792293,
8.61208912631691));
#10984=CARTESIAN_POINT('Ctrl Pts',(-0.669501390402897,0.675208297254384,
8.63253180589755));
#10985=CARTESIAN_POINT('Ctrl Pts',(-0.875992946329232,0.345495322089341,
8.65110259959686));
#10986=CARTESIAN_POINT('Ctrl Pts',(-0.964223900143266,-0.113431902350383,
8.67337382774449));
#10987=CARTESIAN_POINT('Ctrl Pts',(-0.740596150234679,-0.685160402045384,
8.70118563330055));
#10988=CARTESIAN_POINT('Ctrl Pts',(-0.0761424558024043,-1.00505324721318,
8.73452517400358));
#10989=CARTESIAN_POINT('Ctrl Pts',(0.627005912154053,-0.787736452578971,
8.76783232144636));
#10990=CARTESIAN_POINT('Ctrl Pts',(0.994812400535726,-0.150994958894705,
8.80111127518668));
#10991=CARTESIAN_POINT('Ctrl Pts',(0.830981358300232,0.566120360011879,
8.8343664264926));
#10992=CARTESIAN_POINT('Ctrl Pts',(0.325333743617495,0.909742405641226,
8.86206095120001));
#10993=CARTESIAN_POINT('Ctrl Pts',(-0.139139429575983,0.925737554743745,
8.88421060397605));
#10994=CARTESIAN_POINT('Ctrl Pts',(-0.504321857670482,0.798522533185246,
8.90266440172502));
#10995=CARTESIAN_POINT('Ctrl Pts',(-0.813223734583826,0.497308829081565,
8.92295891595097));
#10996=CARTESIAN_POINT('Ctrl Pts',(-0.951958679300059,0.0476855097530266,
8.94509334884795));
#10997=CARTESIAN_POINT('Ctrl Pts',(-0.858568536947436,-0.413287554490503,
8.9672269803888));
#10998=CARTESIAN_POINT('Ctrl Pts',(-0.556269061692827,-0.773731542124292,
8.98935651187958));
#10999=CARTESIAN_POINT('Ctrl Pts',(-0.118502160687732,-0.945376823498998,
9.01148772025747));
#11000=CARTESIAN_POINT('Ctrl Pts',(0.309493444328896,-0.891756529896018,
9.03177362093023));
#11001=CARTESIAN_POINT('Ctrl Pts',(0.636192413112547,-0.685585808620992,
9.05021771711067));
#11002=CARTESIAN_POINT('Ctrl Pts',(0.913553474295901,-0.312947881864283,
9.07235265309009));
#11003=CARTESIAN_POINT('Ctrl Pts',(0.960631698996472,0.296194052975052,
9.10002751178583));
#11004=CARTESIAN_POINT('Ctrl Pts',(0.577840333647451,0.774226230638954,
9.12770811478922));
#11005=CARTESIAN_POINT('Ctrl Pts',(0.138921963035328,0.926247468472041,
9.14986447621748));
#11006=CARTESIAN_POINT('Ctrl Pts',(-0.267314239023255,0.911868754744674,
9.16925630150695));
#11007=CARTESIAN_POINT('Ctrl Pts',(-0.683294438003391,0.682129412884273,
9.19142590162011));
#11008=CARTESIAN_POINT('Ctrl Pts',(-0.941938680245144,0.214161666280006,
9.21638016709812));
#11009=CARTESIAN_POINT('Ctrl Pts',(-0.912098799441386,-0.320403545601203,
9.24134958755738));
#11010=CARTESIAN_POINT('Ctrl Pts',(-0.659446939725027,-0.675689901682901,
9.2617076691118));
#11011=CARTESIAN_POINT('Ctrl Pts',(-0.314783201133364,-0.886337451361902,
9.28115257773485));
#11012=CARTESIAN_POINT('Ctrl Pts',(0.0339048682581715,-0.948027262613349,
9.29782815531288));
#11013=CARTESIAN_POINT('Ctrl Pts',(0.409525764171749,-0.846956944511177,
9.3163673731042));
#11014=CARTESIAN_POINT('Ctrl Pts',(0.691138366917057,-0.639370288018321,
9.33306328330105));
#11015=CARTESIAN_POINT('Ctrl Pts',(0.87750645881461,-0.342726650725962,
9.34976804539523));
#11016=CARTESIAN_POINT('Ctrl Pts',(0.937239721660506,-0.0270902356967322,
9.36509083849118));
#11017=CARTESIAN_POINT('Ctrl Pts',(0.896541377625576,0.259988256337935,
9.37902894066585));
#11018=CARTESIAN_POINT('Ctrl Pts',(0.754698132227089,0.578045031261971,
9.39576347782597));
#11019=CARTESIAN_POINT('Ctrl Pts',(0.420607969490248,0.877087830349221,
9.41669599586192));
#11020=CARTESIAN_POINT('Ctrl Pts',(-0.110985791513677,0.96749605599269,
9.44184448602026));
#11021=CARTESIAN_POINT('Ctrl Pts',(-0.526156759994638,0.795331969305767,
9.46282505153596));
#11022=CARTESIAN_POINT('Ctrl Pts',(-0.765969009939309,0.540947935087001,
9.47962659419499));
#11023=CARTESIAN_POINT('Ctrl Pts',(-0.926993499156135,0.230420411283913,
9.49643868360314));
#11024=CARTESIAN_POINT('Ctrl Pts',(-0.952589676219305,-0.219519434718937,
9.51747248884386));
#11025=CARTESIAN_POINT('Ctrl Pts',(-0.690553452001334,-0.69372499155175,
9.54274789258842));
#11026=CARTESIAN_POINT('Ctrl Pts',(-0.215911709650212,-0.956173277204949,
9.56805844086952));
#11027=CARTESIAN_POINT('Ctrl Pts',(0.326482153616986,-0.925839193894392,
9.59340601342297));
#11028=CARTESIAN_POINT('Ctrl Pts',(0.770238105376938,-0.611104726507316,
9.61879177600974));
#11029=CARTESIAN_POINT('Ctrl Pts',(0.978868207415932,-0.107737371893569,
9.64421717352356));
#11030=CARTESIAN_POINT('Ctrl Pts',(0.887577227206843,0.430343959694922,
9.66968349904293));
#11031=CARTESIAN_POINT('Ctrl Pts',(0.523376342408703,0.838059053917545,
9.6951920503197));
#11032=CARTESIAN_POINT('Ctrl Pts',(-0.00274426362498771,0.989786805195399,
9.72074411643293));
#11033=CARTESIAN_POINT('Ctrl Pts',(-0.530020135210238,0.838080337149508,
9.7463408384755));
#11034=CARTESIAN_POINT('Ctrl Pts',(-0.882514473551932,0.443575823263503,
9.77103386810706));
#11035=CARTESIAN_POINT('Ctrl Pts',(-0.982710426754106,-0.0520415125974364,
9.79481815229705));
#11036=CARTESIAN_POINT('Ctrl Pts',(-0.839404992399888,-0.516361307665272,
9.81769006840781));
#11037=CARTESIAN_POINT('Ctrl Pts',(-0.520010572161815,-0.82826298112752,
9.83869155958704));
#11038=CARTESIAN_POINT('Ctrl Pts',(-0.141709529917495,-0.959945613344496,
9.85781211466694));
#11039=CARTESIAN_POINT('Ctrl Pts',(0.34027152731852,-0.943361696850372,
9.88078772261496));
#11040=CARTESIAN_POINT('Ctrl Pts',(0.7602508065088,-0.658700704986937,9.90380787473997));
#11041=CARTESIAN_POINT('Ctrl Pts',(0.952135045606276,-0.213907148975505,
9.92687574131966));
#11042=CARTESIAN_POINT('Ctrl Pts',(0.971942351738693,0.269920095428384,
9.94997564071361));
#11043=CARTESIAN_POINT('Ctrl Pts',(0.653688535130702,0.82395147603505,9.9789087386129));
#11044=CARTESIAN_POINT('Ctrl Pts',(-0.0826775166361059,1.05146637821754,
10.0137277686201));
#11045=CARTESIAN_POINT('Ctrl Pts',(-0.699434812986587,0.753622187593778,
10.0447664048801));
#11046=CARTESIAN_POINT('Ctrl Pts',(-0.975666081398681,0.244387937000841,
10.0719919503651));
#11047=CARTESIAN_POINT('Ctrl Pts',(-0.975707195393647,-0.252167815721513,
10.0953744497603));
#11048=CARTESIAN_POINT('Ctrl Pts',(-0.737873175341583,-0.689832624733134,
10.1188030808968));
#11049=CARTESIAN_POINT('Ctrl Pts',(-0.318698452927423,-0.960430879264268,
10.1422781619728));
#11050=CARTESIAN_POINT('Ctrl Pts',(0.179821322079405,-0.997802115099903,
10.165801016687));
#11051=CARTESIAN_POINT('Ctrl Pts',(0.569799688583804,-0.821825224718302,
10.1859332990401));
#11052=CARTESIAN_POINT('Ctrl Pts',(0.808529272399683,-0.568786525126624,
10.2026554795479));
#11053=CARTESIAN_POINT('Ctrl Pts',(0.978302334856632,-0.241355508961501,
10.2203816226583));
#11054=CARTESIAN_POINT('Ctrl Pts',(1.00538906456187,0.2333495834722,10.2425768960728));
#11055=CARTESIAN_POINT('Ctrl Pts',(0.728694779250168,0.734236927042486,
10.2692732222169));
#11056=CARTESIAN_POINT('Ctrl Pts',(0.226966011237296,1.01173169163385,10.2960314782446));
#11057=CARTESIAN_POINT('Ctrl Pts',(-0.346931921015741,0.979703466525211,
10.322852197852));
#11058=CARTESIAN_POINT('Ctrl Pts',(-0.816881713892654,0.64646497162191,
10.3497355932434));
#11059=CARTESIAN_POINT('Ctrl Pts',(-1.03804453245733,0.113033933490282,
10.3766819555363));
#11060=CARTESIAN_POINT('Ctrl Pts',(-0.941273337654569,-0.457636831985297,
10.4036914771008));
#11061=CARTESIAN_POINT('Ctrl Pts',(-0.554821661701358,-0.890363150138494,
10.4307643281566));
#11062=CARTESIAN_POINT('Ctrl Pts',(0.0039266343485537,-1.05153545558377,
10.4579006219194));
#11063=CARTESIAN_POINT('Ctrl Pts',(0.56408641499002,-0.890355693773659,
10.4851004304633));
#11064=CARTESIAN_POINT('Ctrl Pts',(0.95354049595536,-0.454843948120234,
10.5123637773334));
#11065=CARTESIAN_POINT('Ctrl Pts',(1.05182093126769,0.122456968256553,10.5396906391692));
#11066=CARTESIAN_POINT('Ctrl Pts',(0.827373278245085,0.664814101527569,
10.5670809495482));
#11067=CARTESIAN_POINT('Ctrl Pts',(0.347668418055166,1.00541156633213,10.5945345871301));
#11068=CARTESIAN_POINT('Ctrl Pts',(-0.241071265795766,1.03865810273544,
10.622051404586));
#11069=CARTESIAN_POINT('Ctrl Pts',(-0.758443515163291,0.752928057938471,
10.6496311647854));
#11070=CARTESIAN_POINT('Ctrl Pts',(-1.04515215340155,0.234550923711717,
10.6772736879972));
#11071=CARTESIAN_POINT('Ctrl Pts',(-1.01205642652925,-0.35823601679832,
10.704978520474));
#11072=CARTESIAN_POINT('Ctrl Pts',(-0.66789446460778,-0.843672061466428,
10.7327456863726));
#11073=CARTESIAN_POINT('Ctrl Pts',(-0.11702199962579,-1.07205102198006,
10.7605740118105));
#11074=CARTESIAN_POINT('Ctrl Pts',(0.472188983917981,-0.972273573004842,
10.7884648797228));
#11075=CARTESIAN_POINT('Ctrl Pts',(0.91890408267479,-0.573161580699387,
10.8164138322953));
#11076=CARTESIAN_POINT('Ctrl Pts',(1.02972492095809,-0.189114130706034,
10.8350920076366));
#11077=CARTESIAN_POINT('Ctrl Pts',(1.02975090409547,0.00389522410502781,
10.8444331682177));
#11078=CARTESIAN_POINT('Ctrl Pts',(1.03719645688851,-0.0037293349184744,
7.95215989910766));
#11079=CARTESIAN_POINT('Ctrl Pts',(1.03717028584552,0.190675813657207,7.96156861253759));
#11080=CARTESIAN_POINT('Ctrl Pts',(0.925557950139338,0.577535603721514,
7.98038266347121));
#11081=CARTESIAN_POINT('Ctrl Pts',(0.475545581675125,0.979605390126322,
8.00853780142747));
#11082=CARTESIAN_POINT('Ctrl Pts',(-0.118073456635005,1.08013597304276,
8.03663686932194));
#11083=CARTESIAN_POINT('Ctrl Pts',(-0.67312151375956,0.850028585888234,
8.06467548649113));
#11084=CARTESIAN_POINT('Ctrl Pts',(-1.01992165763532,0.360873298516457,
8.09265479891218));
#11085=CARTESIAN_POINT('Ctrl Pts',(-1.05327498416264,-0.236503717327239,
8.12057352562096));
#11086=CARTESIAN_POINT('Ctrl Pts',(-0.764326765396757,-0.758933398467517,
8.14843151942941));
#11087=CARTESIAN_POINT('Ctrl Pts',(-0.24287688627644,-1.04691794387519,
8.17622817905231));
#11088=CARTESIAN_POINT('Ctrl Pts',(0.350539555856497,-1.01340964671441,
8.20396316269724));
#11089=CARTESIAN_POINT('Ctrl Pts',(0.834083805209005,-0.670091304275385,
8.23163607534286));
#11090=CARTESIAN_POINT('Ctrl Pts',(1.06033935713661,-0.123370274675711,
8.25924660824643));
#11091=CARTESIAN_POINT('Ctrl Pts',(0.961271344301675,0.458596094063279,
8.28679447706705));
#11092=CARTESIAN_POINT('Ctrl Pts',(0.568649593858113,0.89765324776651,8.31427945443487));
#11093=CARTESIAN_POINT('Ctrl Pts',(0.0039431239572611,1.06012773827784,
8.34170134991208));
#11094=CARTESIAN_POINT('Ctrl Pts',(-0.559405334450464,0.897668914802851,
8.36906003124174));
#11095=CARTESIAN_POINT('Ctrl Pts',(-0.9344966664178,0.477459366698196,8.39534445047533));
#11096=CARTESIAN_POINT('Ctrl Pts',(-1.02319118570897,0.0361130383904124,
8.41652764356969));
#11097=CARTESIAN_POINT('Ctrl Pts',(-0.972095066647408,-0.252162816722124,
8.43062781257449));
#11098=CARTESIAN_POINT('Ctrl Pts',(-0.913310980160994,-0.40757250314265,
8.43867876960068));
#11099=CARTESIAN_POINT('Ctrl Pts',(-0.796998155287066,-0.627946628775765,
8.45074896302428));
#11100=CARTESIAN_POINT('Ctrl Pts',(-0.5220491698584,-0.896088884437607,
8.46883099651776));
#11101=CARTESIAN_POINT('Ctrl Pts',(-0.0296099107857316,-1.03488745726812,
8.49289019054928));
#11102=CARTESIAN_POINT('Ctrl Pts',(0.467306135314492,-0.920636354183639,
8.516899481238));
#11103=CARTESIAN_POINT('Ctrl Pts',(0.913883301313135,-0.528332204193271,
8.54485233012596));
#11104=CARTESIAN_POINT('Ctrl Pts',(1.07128001712609,0.1578675794943,8.57671607247633));
#11105=CARTESIAN_POINT('Ctrl Pts',(0.718979530768331,0.764750753676088,
8.60848123379351));
#11106=CARTESIAN_POINT('Ctrl Pts',(0.181072046006281,1.00590047741433,8.63620356340674));
#11107=CARTESIAN_POINT('Ctrl Pts',(-0.321113972152043,0.968286917313835,
8.65991664175283));
#11108=CARTESIAN_POINT('Ctrl Pts',(-0.708570956654293,0.717751349650519,
8.68160963014022));
#11109=CARTESIAN_POINT('Ctrl Pts',(-0.927415223878402,0.368253958999767,
8.70129511507728));
#11110=CARTESIAN_POINT('Ctrl Pts',(-1.02080929264471,-0.117772384129308,
8.72488167062357));
#11111=CARTESIAN_POINT('Ctrl Pts',(-0.784094990025882,-0.722349424629435,
8.75429895428144));
#11112=CARTESIAN_POINT('Ctrl Pts',(-0.0826159953470804,-1.05973861779947,
8.78949320300836));
#11113=CARTESIAN_POINT('Ctrl Pts',(0.657991980809365,-0.830533515786699,
8.82458319261689));
#11114=CARTESIAN_POINT('Ctrl Pts',(1.04435983522905,-0.161028240208566,
8.85957047777063));
#11115=CARTESIAN_POINT('Ctrl Pts',(0.872191510918413,0.591096145520318,
8.89445647423708));
#11116=CARTESIAN_POINT('Ctrl Pts',(0.342833637985558,0.950500175170697,
8.92344635583295));
#11117=CARTESIAN_POINT('Ctrl Pts',(-0.14240681866231,0.967149549215652,
8.94658832164588));
#11118=CARTESIAN_POINT('Ctrl Pts',(-0.523468734534486,0.83435343134501,
8.96584682092899));
#11119=CARTESIAN_POINT('Ctrl Pts',(-0.845308154191094,0.520393139588824,
8.98699752602333));
#11120=CARTESIAN_POINT('Ctrl Pts',(-0.989543012390118,0.0525630321306637,
9.01003011003576));
#11121=CARTESIAN_POINT('Ctrl Pts',(-0.892450536231069,-0.426209645755978,
9.03302022621514));
#11122=CARTESIAN_POINT('Ctrl Pts',(-0.578881824747128,-0.799912768402463,
9.05597195626933));
#11123=CARTESIAN_POINT('Ctrl Pts',(-0.125687474439124,-0.977501797786432,
9.07888255350409));
#11124=CARTESIAN_POINT('Ctrl Pts',(0.316605904211817,-0.92198833082841,
9.09984979011061));
#11125=CARTESIAN_POINT('Ctrl Pts',(0.653671319469926,-0.709225736145728,
9.11888250352145));
#11126=CARTESIAN_POINT('Ctrl Pts',(0.939439239276747,-0.325183836095085,
9.14169385358281));
#11127=CARTESIAN_POINT('Ctrl Pts',(0.987547025680681,0.301278408095195,
9.17015565689872));
#11128=CARTESIAN_POINT('Ctrl Pts',(0.594679321542008,0.791379583113645,
9.19855495717846));
#11129=CARTESIAN_POINT('Ctrl Pts',(0.145457247238317,0.946900230408442,
9.22123290378143));
#11130=CARTESIAN_POINT('Ctrl Pts',(-0.269744512554461,0.932152140919955,
9.24105448849287));
#11131=CARTESIAN_POINT('Ctrl Pts',(-0.694101106221571,0.697615963332633,
9.26367797146862));
#11132=CARTESIAN_POINT('Ctrl Pts',(-0.957289766597392,0.221074138858957,
9.28908905057342));
#11133=CARTESIAN_POINT('Ctrl Pts',(-0.926805285883287,-0.322025406634136,
9.3144611162));
#11134=CARTESIAN_POINT('Ctrl Pts',(-0.670552563620864,-0.682150076663051,
9.33510504039983));
#11135=CARTESIAN_POINT('Ctrl Pts',(-0.321671655798842,-0.895341345847391,
9.35478847828045));
#11136=CARTESIAN_POINT('Ctrl Pts',(0.0307752103413157,-0.957613220501112,
9.37164419348245));
#11137=CARTESIAN_POINT('Ctrl Pts',(0.409786204776528,-0.855569172091428,
9.39035412038357));
#11138=CARTESIAN_POINT('Ctrl Pts',(0.693500977439743,-0.646372437096977,
9.40717726375736));
#11139=CARTESIAN_POINT('Ctrl Pts',(0.880977325954236,-0.347876678883315,
9.42398736672525));
#11140=CARTESIAN_POINT('Ctrl Pts',(0.940946228891237,-0.0307571479885627,
9.43938348179057));
#11141=CARTESIAN_POINT('Ctrl Pts',(0.900090933330989,0.257284228276144,
9.45336988898821));
#11142=CARTESIAN_POINT('Ctrl Pts',(0.75789942871261,0.576053653419727,9.47014345990121));
#11143=CARTESIAN_POINT('Ctrl Pts',(0.423486133635302,0.87520526392437,9.49109488900207));
#11144=CARTESIAN_POINT('Ctrl Pts',(-0.107317293259283,0.965309921368965,
9.51620779009144));
#11145=CARTESIAN_POINT('Ctrl Pts',(-0.520902213846082,0.793666918986136,
9.53711515836644));
#11146=CARTESIAN_POINT('Ctrl Pts',(-0.759397793029819,0.54064129614791,
9.55382724163822));
#11147=CARTESIAN_POINT('Ctrl Pts',(-0.919357990870187,0.232108695129427,
9.57053164436102));
#11148=CARTESIAN_POINT('Ctrl Pts',(-0.944612254049654,-0.214222806773856,
9.59140013603058));
#11149=CARTESIAN_POINT('Ctrl Pts',(-0.685107321886509,-0.683500930880567,
9.61642055252469));
#11150=CARTESIAN_POINT('Ctrl Pts',(-0.216252770756576,-0.942567517453279,
9.6414222205253));
#11151=CARTESIAN_POINT('Ctrl Pts',(0.318278561645482,-0.912511970668242,
9.66640623507196));
#11152=CARTESIAN_POINT('Ctrl Pts',(0.754581459699137,-0.602868595837562,
9.69137453525599));
#11153=CARTESIAN_POINT('Ctrl Pts',(0.959169418745129,-0.108840250447074,
9.7163286998096));
#11154=CARTESIAN_POINT('Ctrl Pts',(0.869615683384371,0.418055869863705,
9.74127046801076));
#11155=CARTESIAN_POINT('Ctrl Pts',(0.513593683823807,0.816378372045758,
9.7662015614447));
#11156=CARTESIAN_POINT('Ctrl Pts',(0.000472864523384456,0.964194355862096,
9.7911236329607));
#11157=CARTESIAN_POINT('Ctrl Pts',(-0.512639156114366,0.816398384562372,
9.8160385797356));
#11158=CARTESIAN_POINT('Ctrl Pts',(-0.854897593072207,0.433135404547336,
9.84002524516739));
#11159=CARTESIAN_POINT('Ctrl Pts',(-0.951920813198652,-0.0473618249043272,
9.86308637136708));
#11160=CARTESIAN_POINT('Ctrl Pts',(-0.813150828637682,-0.496663759626729,
9.8852216709568));
#11161=CARTESIAN_POINT('Ctrl Pts',(-0.504527693025104,-0.797911067211824,
9.90551184440933));
#11162=CARTESIAN_POINT('Ctrl Pts',(-0.139592336256419,-0.924897874793092,
9.9239588016233));
#11163=CARTESIAN_POINT('Ctrl Pts',(0.32476002062656,-0.908862355890077,
9.94609483836991));
#11164=CARTESIAN_POINT('Ctrl Pts',(0.728526143184254,-0.634941072206952,
9.96823570550932));
#11165=CARTESIAN_POINT('Ctrl Pts',(0.912651243172658,-0.207993974856502,
9.9903798965011));
#11166=CARTESIAN_POINT('Ctrl Pts',(0.93159093211479,0.255865599740591,10.0125272672192));
#11167=CARTESIAN_POINT('Ctrl Pts',(0.626775516099417,0.785983302959022,
10.0402233323282));
#11168=CARTESIAN_POINT('Ctrl Pts',(-0.0764260103068494,1.00290823265387,
10.0734741130373));
#11169=CARTESIAN_POINT('Ctrl Pts',(-0.663913049810778,0.718917831796266,
10.1030507684028));
#11170=CARTESIAN_POINT('Ctrl Pts',(-0.926512975578048,0.234583456765021,
10.1289456687419));
#11171=CARTESIAN_POINT('Ctrl Pts',(-0.926479271132153,-0.236978839253667,
10.1511526887213));
#11172=CARTESIAN_POINT('Ctrl Pts',(-0.700839853017446,-0.652019794966121,
10.1733738737333));
#11173=CARTESIAN_POINT('Ctrl Pts',(-0.303776802726922,-0.908251612454935,
10.1956106345133));
#11174=CARTESIAN_POINT('Ctrl Pts',(0.167783237861881,-0.943528965310917,
10.2178619614777));
#11175=CARTESIAN_POINT('Ctrl Pts',(0.536202295862543,-0.777216710409037,
10.2368850275763));
#11176=CARTESIAN_POINT('Ctrl Pts',(0.76151294157343,-0.538381201717669,
10.2526688564185));
#11177=CARTESIAN_POINT('Ctrl Pts',(0.921632025245598,-0.229535734594294,
10.2693891391398));
#11178=CARTESIAN_POINT('Ctrl Pts',(0.947080496251134,0.217794926170324,
10.2903068420048));
#11179=CARTESIAN_POINT('Ctrl Pts',(0.686598901099996,0.689141902373008,
10.3154333425304));
#11180=CARTESIAN_POINT('Ctrl Pts',(0.214945265052869,0.94990696216286,10.3405880336628));
#11181=CARTESIAN_POINT('Ctrl Pts',(-0.323876018866969,0.919752968003473,
10.3657719058747));
#11182=CARTESIAN_POINT('Ctrl Pts',(-0.764572616499986,0.607160410323047,
10.3909867552046));
#11183=CARTESIAN_POINT('Ctrl Pts',(-0.971702406404501,0.107377544455468,
10.4162339680835));
#11184=CARTESIAN_POINT('Ctrl Pts',(-0.881059610722316,-0.426720480341076,
10.4415150769132));
#11185=CARTESIAN_POINT('Ctrl Pts',(-0.519655694997322,-0.831297350140601,
10.4668315108411));
#11186=CARTESIAN_POINT('Ctrl Pts',(0.00235883360422653,-0.98180710952777,
10.4921846931895));
#11187=CARTESIAN_POINT('Ctrl Pts',(0.525223150865608,-0.831296672923994,
10.5175760215671));
#11188=CARTESIAN_POINT('Ctrl Pts',(0.888435991055881,-0.425046664919749,
10.5430068558293));
#11189=CARTESIAN_POINT('Ctrl Pts',(0.979988661732392,0.113038466202106,
10.5684785338995));
#11190=CARTESIAN_POINT('Ctrl Pts',(0.770886513678643,0.618192706747942,
10.5939923551312));
#11191=CARTESIAN_POINT('Ctrl Pts',(0.324317244435882,0.935211426154897,
10.6195495969629));
#11192=CARTESIAN_POINT('Ctrl Pts',(-0.22342646197345,0.966104184880575,
10.6451514997004));
#11193=CARTESIAN_POINT('Ctrl Pts',(-0.704517100257862,0.700372287633452,
10.6707992716954));
#11194=CARTESIAN_POINT('Ctrl Pts',(-0.970986492881063,0.218523865304527,
10.6964940855284));
#11195=CARTESIAN_POINT('Ctrl Pts',(-0.940209380211664,-0.332262593742652,
10.7222371038369));
#11196=CARTESIAN_POINT('Ctrl Pts',(-0.620514508604514,-0.783155463378012,
10.7480293919687));
#11197=CARTESIAN_POINT('Ctrl Pts',(-0.10896221887375,-0.995208970605426,
10.7738721348519));
#11198=CARTESIAN_POINT('Ctrl Pts',(0.43807428354937,-0.902589090530947,
10.7997661462395));
#11199=CARTESIAN_POINT('Ctrl Pts',(0.85274473405393,-0.532059372519866,
10.8257129556942));
#11200=CARTESIAN_POINT('Ctrl Pts',(0.955606232646419,-0.175711702508772,
10.8430448118064));
#11201=CARTESIAN_POINT('Ctrl Pts',(0.955630365396176,0.00355250229995129,
10.8517207421788));
#11202=CARTESIAN_POINT('Ctrl Pts',(1.0838482003043,-0.000914448548792532,
7.89412779065783));
#11203=CARTESIAN_POINT('Ctrl Pts',(1.08382086259523,0.202156991753356,7.90395593050703));
#11204=CARTESIAN_POINT('Ctrl Pts',(0.96716342125297,0.606732997046235,7.92363301940144));
#11205=CARTESIAN_POINT('Ctrl Pts',(0.496000875527845,1.02784680220822,7.95311729373211));
#11206=CARTESIAN_POINT('Ctrl Pts',(-0.126541219357233,1.13341877234435,
7.98258888834162));
#11207=CARTESIAN_POINT('Ctrl Pts',(-0.709545608469748,0.891862572219048,
8.01203898822628));
#11208=CARTESIAN_POINT('Ctrl Pts',(-1.07441005641409,0.377463005767994,
8.04146921435643));
#11209=CARTESIAN_POINT('Ctrl Pts',(-1.10966865400436,-0.251710046816853,
8.07087652363246));
#11210=CARTESIAN_POINT('Ctrl Pts',(-0.805032466753758,-0.80276307880036,
8.10025997100121));
#11211=CARTESIAN_POINT('Ctrl Pts',(-0.254398208228186,-1.10700349947945,
8.12961768909314));
#11212=CARTESIAN_POINT('Ctrl Pts',(0.373117719641826,-1.07168631577933,
8.15894823924168));
#11213=CARTESIAN_POINT('Ctrl Pts',(0.88515438734053,-0.708276627835562,
8.18825002300904));
#11214=CARTESIAN_POINT('Ctrl Pts',(1.12510635980224,-0.128745368292323,
8.21752154423205));
#11215=CARTESIAN_POINT('Ctrl Pts',(1.02006457029756,0.488942832092543,8.24676128145543));
#11216=CARTESIAN_POINT('Ctrl Pts',(0.602951017257973,0.95554132784791,8.27596778161598));
#11217=CARTESIAN_POINT('Ctrl Pts',(0.00226783791176727,1.12846883942168,
8.30513956604923));
#11218=CARTESIAN_POINT('Ctrl Pts',(-0.597667353003912,0.955557647790115,
8.33427528667529));
#11219=CARTESIAN_POINT('Ctrl Pts',(-0.997580811393811,0.507673638651765,
8.36229572045689));
#11220=CARTESIAN_POINT('Ctrl Pts',(-1.09227219135141,0.0367679381382032,
8.38489914841893));
#11221=CARTESIAN_POINT('Ctrl Pts',(-1.03772824844162,-0.271014548929116,
8.39995360230054));
#11222=CARTESIAN_POINT('Ctrl Pts',(-0.974949204552547,-0.436989591216038,
8.40855194537982));
#11223=CARTESIAN_POINT('Ctrl Pts',(-0.850705795757624,-0.672393715416174,
8.42144546139659));
#11224=CARTESIAN_POINT('Ctrl Pts',(-0.556878890231008,-0.959006027648614,
8.44077179267571));
#11225=CARTESIAN_POINT('Ctrl Pts',(-0.0301913926151124,-1.10751276767793,
8.46650528584973));
#11226=CARTESIAN_POINT('Ctrl Pts',(0.501708333376544,-0.98527102028979,
8.49220475204497));
#11227=CARTESIAN_POINT('Ctrl Pts',(0.980083971872979,-0.565112204961699,
8.52214616157649));
#11228=CARTESIAN_POINT('Ctrl Pts',(1.14895607407238,0.170475723569411,8.55630580617952));
#11229=CARTESIAN_POINT('Ctrl Pts',(0.7710459574588,0.821732127342494,8.59039054363123));
#11230=CARTESIAN_POINT('Ctrl Pts',(0.193487242513833,1.08070806313451,8.62015730147285));
#11231=CARTESIAN_POINT('Ctrl Pts',(-0.346009171336449,1.04033345516453,
8.64563214466693));
#11232=CARTESIAN_POINT('Ctrl Pts',(-0.762466515394437,0.771083934602891,
8.66894777270452));
#11233=CARTESIAN_POINT('Ctrl Pts',(-0.99778215525873,0.395306289766034,
8.69011375490029));
#11234=CARTESIAN_POINT('Ctrl Pts',(-1.0982483309166,-0.127426784513864,
8.71548185859923));
#11235=CARTESIAN_POINT('Ctrl Pts',(-0.843613153081136,-0.777967142474131,
8.74713381288415));
#11236=CARTESIAN_POINT('Ctrl Pts',(-0.088507342272469,-1.14122962611758,
8.78501928785707));
#11237=CARTESIAN_POINT('Ctrl Pts',(0.709065757260984,-0.894452196565483,
8.82280637288963));
#11238=CARTESIAN_POINT('Ctrl Pts',(1.12529561032464,-0.173286632271806,
8.86049290545786));
#11239=CARTESIAN_POINT('Ctrl Pts',(0.939827863300308,0.637049421449346,
8.89807721520378));
#11240=CARTESIAN_POINT('Ctrl Pts',(0.369468399528226,1.02430481692951,8.92931078741886));
#11241=CARTESIAN_POINT('Ctrl Pts',(-0.15336583993037,1.0422444816976,8.95424500292052));
#11242=CARTESIAN_POINT('Ctrl Pts',(-0.563936805331798,0.899166803592543,
8.97499399053462));
#11243=CARTESIAN_POINT('Ctrl Pts',(-0.910669570745192,0.560918417615995,
8.99777978341788));
#11244=CARTESIAN_POINT('Ctrl Pts',(-1.06604101086678,0.0569636584812059,
9.02258893664379));
#11245=CARTESIAN_POINT('Ctrl Pts',(-0.961451537401035,-0.458702011613492,
9.0473503347936));
#11246=CARTESIAN_POINT('Ctrl Pts',(-0.623794994012935,-0.861102456908409,
9.0720625968117));
#11247=CARTESIAN_POINT('Ctrl Pts',(-0.135894920546228,-1.05227024528694,
9.0967266248224));
#11248=CARTESIAN_POINT('Ctrl Pts',(0.340102284602575,-0.992509712058549,
9.11928978647568));
#11249=CARTESIAN_POINT('Ctrl Pts',(0.702746144635939,-0.763590236431144,
9.13976608516106));
#11250=CARTESIAN_POINT('Ctrl Pts',(1.01011084241462,-0.350500037079963,
9.16430047463988));
#11251=CARTESIAN_POINT('Ctrl Pts',(1.0617514972005,0.323027753091657,9.19489901500147));
#11252=CARTESIAN_POINT('Ctrl Pts',(0.639624221556973,0.84946830932992,9.22540199762321));
#11253=CARTESIAN_POINT('Ctrl Pts',(0.157300877416754,1.01642810811852,9.24974966923183));
#11254=CARTESIAN_POINT('Ctrl Pts',(-0.288301982182871,1.00058338021818,
9.27102081642107));
#11255=CARTESIAN_POINT('Ctrl Pts',(-0.743430664340233,0.74898609481149,
9.29528306623843));
#11256=CARTESIAN_POINT('Ctrl Pts',(-1.02546174642978,0.238215657258133,
9.32251462671953));
#11257=CARTESIAN_POINT('Ctrl Pts',(-0.992748476251999,-0.343390555439158,
9.34968277653113));
#11258=CARTESIAN_POINT('Ctrl Pts',(-0.718527463530067,-0.728675713878542,
9.37176741485846));
#11259=CARTESIAN_POINT('Ctrl Pts',(-0.345458809407523,-0.956634300940651,
9.39281388741142));
#11260=CARTESIAN_POINT('Ctrl Pts',(0.0311884895998242,-1.02314357299083,
9.41082562368356));
#11261=CARTESIAN_POINT('Ctrl Pts',(0.435880506281094,-0.914158731694693,
9.43080150015021));
#11262=CARTESIAN_POINT('Ctrl Pts',(0.738620974493306,-0.690909070523313,
9.44875254494689));
#11263=CARTESIAN_POINT('Ctrl Pts',(0.9385024099283,-0.372611741600812,9.46667467159655));
#11264=CARTESIAN_POINT('Ctrl Pts',(1.00237872112136,-0.0347073992703695,
9.48307805826784));
#11265=CARTESIAN_POINT('Ctrl Pts',(0.958861569486603,0.272010577946869,
9.49797018640025));
#11266=CARTESIAN_POINT('Ctrl Pts',(0.807519793645455,0.611255165848026,
9.51582019885214));
#11267=CARTESIAN_POINT('Ctrl Pts',(0.451909976937506,0.929265184877128,
9.53809184874244));
#11268=CARTESIAN_POINT('Ctrl Pts',(-0.111797110794033,1.0248480893635,9.56475740718536));
#11269=CARTESIAN_POINT('Ctrl Pts',(-0.550390920642296,0.842725120389943,
9.58692643984169));
#11270=CARTESIAN_POINT('Ctrl Pts',(-0.803077343857937,0.574617344448347,
9.60463278999863));
#11271=CARTESIAN_POINT('Ctrl Pts',(-0.97243696867917,0.247916429508408,
9.62231887693885));
#11272=CARTESIAN_POINT('Ctrl Pts',(-0.999058693555682,-0.224167470527981,
9.64438690207702));
#11273=CARTESIAN_POINT('Ctrl Pts',(-0.724871986515919,-0.719760375599744,
9.6708095787426));
#11274=CARTESIAN_POINT('Ctrl Pts',(-0.230348354153974,-0.992872189570322,
9.69717262938872));
#11275=CARTESIAN_POINT('Ctrl Pts',(0.332515958586368,-0.961100479168014,
9.72347720468563));
#11276=CARTESIAN_POINT('Ctrl Pts',(0.791156172152085,-0.635448799884614,
9.74972373646253));
#11277=CARTESIAN_POINT('Ctrl Pts',(1.00578640215473,-0.116833985348966,
9.77591303739745));
#11278=CARTESIAN_POINT('Ctrl Pts',(0.911811450066463,0.435293222025004,
9.80204583327431));
#11279=CARTESIAN_POINT('Ctrl Pts',(0.539261434877731,0.851908601823872,
9.82812290732319));
#11280=CARTESIAN_POINT('Ctrl Pts',(0.00336028235764251,1.00614792986501,
9.85414516087386));
#11281=CARTESIAN_POINT('Ctrl Pts',(-0.531503227958469,0.851946292011022,
9.88011328551953));
#11282=CARTESIAN_POINT('Ctrl Pts',(-0.887541808641719,0.453048239768111,
9.90506874294698));
#11283=CARTESIAN_POINT('Ctrl Pts',(-0.988224862711454,-0.0460782804447304,
9.92901840717504));
#11284=CARTESIAN_POINT('Ctrl Pts',(-0.844211613760868,-0.511992487885777,
9.95197147120267));
#11285=CARTESIAN_POINT('Ctrl Pts',(-0.52463839039403,-0.823802817820016,
9.9729753411795));
#11286=CARTESIAN_POINT('Ctrl Pts',(-0.147402040593785,-0.955022699264225,
9.99204031078243));
#11287=CARTESIAN_POINT('Ctrl Pts',(0.331994552727527,-0.938394674293537,
10.0148912553923));
#11288=CARTESIAN_POINT('Ctrl Pts',(0.747859600288323,-0.655983436748773,
10.0376971514725));
#11289=CARTESIAN_POINT('Ctrl Pts',(0.937105692798899,-0.216960017735763,
10.0604636979959));
#11290=CARTESIAN_POINT('Ctrl Pts',(0.956494142862348,0.259388583755504,
10.0832041717988));
#11291=CARTESIAN_POINT('Ctrl Pts',(0.643862373212363,0.802456461011887,
10.1115758852511));
#11292=CARTESIAN_POINT('Ctrl Pts',(-0.0748631700336077,1.02374906025246,
10.1455482688799));
#11293=CARTESIAN_POINT('Ctrl Pts',(-0.673362689405438,0.734057071294702,
10.1756792735207));
#11294=CARTESIAN_POINT('Ctrl Pts',(-0.940211173985656,0.241612490483782,
10.2020001217299));
#11295=CARTESIAN_POINT('Ctrl Pts',(-0.940061131273621,-0.236900273902396,
10.2245322988002));
#11296=CARTESIAN_POINT('Ctrl Pts',(-0.711446123935283,-0.657195553614125,
10.247034622298));
#11297=CARTESIAN_POINT('Ctrl Pts',(-0.310032668855504,-0.916099462990559,
10.2695077971124));
#11298=CARTESIAN_POINT('Ctrl Pts',(0.165734041548867,-0.951573099062055,
10.291955877611));
#11299=CARTESIAN_POINT('Ctrl Pts',(0.536637465797884,-0.78402716349881,
10.311104963167));
#11300=CARTESIAN_POINT('Ctrl Pts',(0.76314851915361,-0.543880336389376,
10.3269730190361));
#11301=CARTESIAN_POINT('Ctrl Pts',(0.923937995332574,-0.233678441944692,
10.3437641472873));
#11302=CARTESIAN_POINT('Ctrl Pts',(0.949313105102571,0.214827832547124,
10.3647313433219));
#11303=CARTESIAN_POINT('Ctrl Pts',(0.688565919279137,0.686304166961507,
10.389864829251));
#11304=CARTESIAN_POINT('Ctrl Pts',(0.217650841892384,0.946463195692629,
10.4149706945773));
#11305=CARTESIAN_POINT('Ctrl Pts',(-0.319048217451104,0.916258727218333,
10.440051304975));
#11306=CARTESIAN_POINT('Ctrl Pts',(-0.756961259842281,0.605434323983068,
10.4651078480003));
#11307=CARTESIAN_POINT('Ctrl Pts',(-0.962226484778156,0.109716966678491,
10.4901420759625));
#11308=CARTESIAN_POINT('Ctrl Pts',(-0.872365348998548,-0.418790659164996,
10.5151555282894));
#11309=CARTESIAN_POINT('Ctrl Pts',(-0.515377026932851,-0.818178757886243,
10.5401498745057));
#11310=CARTESIAN_POINT('Ctrl Pts',(-0.000980240333085043,-0.966322769852347,
10.5651267379984));
#11311=CARTESIAN_POINT('Ctrl Pts',(0.513063068024907,-0.818183101349432,
10.5900878010138));
#11312=CARTESIAN_POINT('Ctrl Pts',(0.869301976324407,-0.419491985735566,
10.6150347288481));
#11313=CARTESIAN_POINT('Ctrl Pts',(0.958780479694553,0.1073556061531,10.6399692179751));
#11314=CARTESIAN_POINT('Ctrl Pts',(0.754335676381123,0.600843600178277,
10.6648929541654));
#11315=CARTESIAN_POINT('Ctrl Pts',(0.318834621372516,0.90981229213662,10.6898076577536));
#11316=CARTESIAN_POINT('Ctrl Pts',(-0.214141831829799,0.939716543474692,
10.7147150160685));
#11317=CARTESIAN_POINT('Ctrl Pts',(-0.681238257715304,0.68154065932501,
10.7396167908086));
#11318=CARTESIAN_POINT('Ctrl Pts',(-0.939353232681883,0.214492092469083,
10.7645145830463));
#11319=CARTESIAN_POINT('Ctrl Pts',(-0.909441174443961,-0.318236929963865,
10.7894103781415));
#11320=CARTESIAN_POINT('Ctrl Pts',(-0.600708513133185,-0.753434977070502,
10.8143052762627));
#11321=CARTESIAN_POINT('Ctrl Pts',(-0.107767289636025,-0.957617587334566,
10.8392023443988));
#11322=CARTESIAN_POINT('Ctrl Pts',(0.418292015354745,-0.868431439290108,
10.8641002181391));
#11323=CARTESIAN_POINT('Ctrl Pts',(0.816252889411692,-0.512592296203714,
10.8890073890965));
#11324=CARTESIAN_POINT('Ctrl Pts',(0.914688282568999,-0.171209962575356,
10.9056065352154));
#11325=CARTESIAN_POINT('Ctrl Pts',(0.914711404788378,0.000547765501091019,
10.9139191712561));
#11326=CARTESIAN_POINT('Ctrl Pts',(1.06701743632438,0.0025960290114382,
7.82154662476291));
#11327=CARTESIAN_POINT('Ctrl Pts',(1.06699050603538,0.202641049598823,7.83122829361572));
#11328=CARTESIAN_POINT('Ctrl Pts',(0.952169403602462,0.601316966034855,
7.850613547215));
#11329=CARTESIAN_POINT('Ctrl Pts',(0.487093861785577,1.01725013287211,7.87972343428257));
#11330=CARTESIAN_POINT('Ctrl Pts',(-0.128666178509213,1.12181753997798,
7.90887159798562));
#11331=CARTESIAN_POINT('Ctrl Pts',(-0.706490994785343,0.882579858430546,
7.93805444725339));
#11332=CARTESIAN_POINT('Ctrl Pts',(-1.06888045229236,0.371930676583893,
7.96727152805071));
#11333=CARTESIAN_POINT('Ctrl Pts',(-1.10411045676727,-0.253923420995056,
7.99652093475803));
#11334=CARTESIAN_POINT('Ctrl Pts',(-0.800647763134568,-0.803185289622725,
8.02580137401769));
#11335=CARTESIAN_POINT('Ctrl Pts',(-0.250930641224358,-1.10710470404373,
8.05511124460616));
#11336=CARTESIAN_POINT('Ctrl Pts',(0.376814540590657,-1.07193905643761,
8.08444904323414));
#11337=CARTESIAN_POINT('Ctrl Pts',(0.890086824381486,-0.707854158546105,
8.11381319934604));
#11338=CARTESIAN_POINT('Ctrl Pts',(1.13117627450501,-0.126006039541308,
8.14320213996355));
#11339=CARTESIAN_POINT('Ctrl Pts',(1.02566796039198,0.495407813750173,8.17261426104031));
#11340=CARTESIAN_POINT('Ctrl Pts',(0.605395747600651,0.965787356705992,
8.20204794473113));
#11341=CARTESIAN_POINT('Ctrl Pts',(-0.00109610972165227,1.14055805748304,
8.2315015642435));
#11342=CARTESIAN_POINT('Ctrl Pts',(-0.608048139592871,0.965796133351913,
8.26097343779502));
#11343=CARTESIAN_POINT('Ctrl Pts',(-1.01347415035759,0.51197072632285,8.28936978311824));
#11344=CARTESIAN_POINT('Ctrl Pts',(-1.10970380118711,0.033896466150247,
8.31231621328207));
#11345=CARTESIAN_POINT('Ctrl Pts',(-1.05427292616554,-0.27897678633527,
8.32761884188052));
#11346=CARTESIAN_POINT('Ctrl Pts',(-0.990418366398432,-0.447799765271943,
8.33636455425477));
#11347=CARTESIAN_POINT('Ctrl Pts',(-0.863997036800892,-0.68734004421506,
8.34948431630875));
#11348=CARTESIAN_POINT('Ctrl Pts',(-0.56477516495449,-0.97932462816657,
8.3691676579603));
#11349=CARTESIAN_POINT('Ctrl Pts',(-0.0274664722784836,-1.13095114472672,
8.39542113766043));
#11350=CARTESIAN_POINT('Ctrl Pts',(0.516092848385612,-1.00613117413851,
8.42168142940329));
#11351=CARTESIAN_POINT('Ctrl Pts',(1.0057877897569,-0.576213269843886,8.45232537141141));
#11352=CARTESIAN_POINT('Ctrl Pts',(1.17928912153765,0.178065478023402,8.48735422482944));
#11353=CARTESIAN_POINT('Ctrl Pts',(0.791104418082697,0.847685062285886,
8.52238889521533));
#11354=CARTESIAN_POINT('Ctrl Pts',(0.196290711324304,1.11453858289063,8.5530461496888));
#11355=CARTESIAN_POINT('Ctrl Pts',(-0.360219354067838,1.0729904639039,8.5793236664903));
#11356=CARTESIAN_POINT('Ctrl Pts',(-0.790510042128262,0.794916107930365,
8.60341001062862));
#11357=CARTESIAN_POINT('Ctrl Pts',(-1.03397172011655,0.40621012607091,8.62530485816356));
#11358=CARTESIAN_POINT('Ctrl Pts',(-1.13807370548541,-0.135112100279007,
8.65157605998515));
#11359=CARTESIAN_POINT('Ctrl Pts',(-0.874200603918551,-0.810033907036799,
8.68440883732023));
#11360=CARTESIAN_POINT('Ctrl Pts',(-0.0893495425282713,-1.1880032461031,
8.72379427305056));
#11361=CARTESIAN_POINT('Ctrl Pts',(0.741691192429426,-0.931226721392334,
8.76316169471054));
#11362=CARTESIAN_POINT('Ctrl Pts',(1.17652809635137,-0.178488859217621,
8.80250720794144));
#11363=CARTESIAN_POINT('Ctrl Pts',(0.982824576300801,0.669329348618244,
8.84182661196442));
#11364=CARTESIAN_POINT('Ctrl Pts',(0.385078060730947,1.07548591500891,8.87456816417469));
#11365=CARTESIAN_POINT('Ctrl Pts',(-0.163794877304455,1.09437112850357,
8.90074393179308));
#11366=CARTESIAN_POINT('Ctrl Pts',(-0.595227163902899,0.944061642655201,
8.9225472241168));
#11367=CARTESIAN_POINT('Ctrl Pts',(-0.960030174906419,0.588294670681147,
8.94651746619086));
#11368=CARTESIAN_POINT('Ctrl Pts',(-1.12375366033643,0.0575187100594699,
8.97264926310775));
#11369=CARTESIAN_POINT('Ctrl Pts',(-1.01354227711893,-0.486285552237881,
8.99876117296623));
#11370=CARTESIAN_POINT('Ctrl Pts',(-0.65710031907676,-0.911189326968473,
9.02485391772391));
#11371=CARTESIAN_POINT('Ctrl Pts',(-0.141413823150027,-1.11332884259046,
9.05092443890678));
#11372=CARTESIAN_POINT('Ctrl Pts',(0.36230898904362,-1.05015688586155,9.0748027078103));
#11373=CARTESIAN_POINT('Ctrl Pts',(0.746453838137557,-0.807699772902029,
9.09649267546183));
#11374=CARTESIAN_POINT('Ctrl Pts',(1.07231758997464,-0.369824731298935,
9.12250252624746));
#11375=CARTESIAN_POINT('Ctrl Pts',(1.12732730366444,0.345001885129974,9.15497914731887));
#11376=CARTESIAN_POINT('Ctrl Pts',(0.678756713757859,0.904746517993574,
9.18740855014101));
#11377=CARTESIAN_POINT('Ctrl Pts',(0.165507019098447,1.08244751652205,9.21331839979818));
#11378=CARTESIAN_POINT('Ctrl Pts',(-0.308999581863406,1.06560418820654,
9.23597081782354));
#11379=CARTESIAN_POINT('Ctrl Pts',(-0.794117710088271,0.797513049435794,
9.26183226756409));
#11380=CARTESIAN_POINT('Ctrl Pts',(-1.09507393875302,0.252625058546865,
9.29088748480864));
#11381=CARTESIAN_POINT('Ctrl Pts',(-1.06021949391649,-0.368467310983676,
9.31990238809889));
#11382=CARTESIAN_POINT('Ctrl Pts',(-0.767155367175566,-0.780323412962235,
9.34351106352889));
#11383=CARTESIAN_POINT('Ctrl Pts',(-0.368167386477954,-1.02413220651149,
9.36602115249684));
#11384=CARTESIAN_POINT('Ctrl Pts',(0.0348719585901695,-1.09533669341058,
9.38529619984537));
#11385=CARTESIAN_POINT('Ctrl Pts',(0.468219703484827,-0.978655860325924,
9.40668812759201));
#11386=CARTESIAN_POINT('Ctrl Pts',(0.792553898291587,-0.739500371751133,
9.42591990841105));
#11387=CARTESIAN_POINT('Ctrl Pts',(1.00681767370294,-0.398335671185081,
9.44513223986786));
#11388=CARTESIAN_POINT('Ctrl Pts',(1.07533028922252,-0.0359819011052655,
9.46272410868506));
#11389=CARTESIAN_POINT('Ctrl Pts',(1.0286539815297,0.293056390755808,9.47870105477657));
#11390=CARTESIAN_POINT('Ctrl Pts',(0.86625698295483,0.657104215112349,9.49785707208013));
#11391=CARTESIAN_POINT('Ctrl Pts',(0.484475150056015,0.998571613108099,
9.52177366135875));
#11392=CARTESIAN_POINT('Ctrl Pts',(-0.121083850117737,1.10130133263869,
9.55042230310675));
#11393=CARTESIAN_POINT('Ctrl Pts',(-0.592522878860891,0.905583663059082,
9.57425486906399));
#11394=CARTESIAN_POINT('Ctrl Pts',(-0.864209344596109,0.617325533939084,
9.59329337909015));
#11395=CARTESIAN_POINT('Ctrl Pts',(-1.04634541117236,0.265991724838279,
9.6123144658592));
#11396=CARTESIAN_POINT('Ctrl Pts',(-1.07500987210398,-0.24188060268642,
9.63605956488873));
#11397=CARTESIAN_POINT('Ctrl Pts',(-0.779954867934298,-0.775246119869282,
9.66449897772344));
#11398=CARTESIAN_POINT('Ctrl Pts',(-0.247592524130115,-1.06928473269863,
9.69288403823075));
#11399=CARTESIAN_POINT('Ctrl Pts',(0.358514842778508,-1.03509158560357,
9.72121339508318));
#11400=CARTESIAN_POINT('Ctrl Pts',(0.852503408868504,-0.684360220801713,
9.74948648590963));
#11401=CARTESIAN_POINT('Ctrl Pts',(1.08371728012903,-0.125699851986608,
9.77770245803913));
#11402=CARTESIAN_POINT('Ctrl Pts',(0.98247853245713,0.469127299242737,9.80586062858382));
#11403=CARTESIAN_POINT('Ctrl Pts',(0.581095418885572,0.917982863355751,
9.8339603391256));
#11404=CARTESIAN_POINT('Ctrl Pts',(0.00371945698538958,1.0841505904603,
9.86200090585858));
#11405=CARTESIAN_POINT('Ctrl Pts',(-0.572497970703721,0.918009674239079,
9.88998191493704));
#11406=CARTESIAN_POINT('Ctrl Pts',(-0.956015873607097,0.48830415267755,
9.91686840080534));
#11407=CARTESIAN_POINT('Ctrl Pts',(-1.06443510009297,-0.0492810426968473,
9.94266804966375));
#11408=CARTESIAN_POINT('Ctrl Pts',(-0.909357052100821,-0.550964155960349,
9.96738574321015));
#11409=CARTESIAN_POINT('Ctrl Pts',(-0.565311440336517,-0.886619648503672,
9.98999909150709));
#11410=CARTESIAN_POINT('Ctrl Pts',(-0.159295255073405,-1.02784076843099,
10.0105219760513));
#11411=CARTESIAN_POINT('Ctrl Pts',(0.356531087367818,-1.00994129487403,
10.0351110691776));
#11412=CARTESIAN_POINT('Ctrl Pts',(0.803815564251162,-0.70612787785747,
10.0596470195591));
#11413=CARTESIAN_POINT('Ctrl Pts',(1.00725255818897,-0.23415518199599,10.0841256738831));
#11414=CARTESIAN_POINT('Ctrl Pts',(1.02807331078756,0.277760194562661,10.1085663359638));
#11415=CARTESIAN_POINT('Ctrl Pts',(0.692177038145714,0.86105028376297,10.1390509198933));
#11416=CARTESIAN_POINT('Ctrl Pts',(-0.079207548479385,1.09839920332005,
10.1755177213482));
#11417=CARTESIAN_POINT('Ctrl Pts',(-0.720878115552071,0.787669451110676,
10.2078339278888));
#11418=CARTESIAN_POINT('Ctrl Pts',(-1.00668116603609,0.260095185285768,
10.2360361718044));
#11419=CARTESIAN_POINT('Ctrl Pts',(-1.00648111171243,-0.252125402489005,
10.260158097259));
#11420=CARTESIAN_POINT('Ctrl Pts',(-0.761884595208099,-0.70166277460692,
10.2842305712202));
#11421=CARTESIAN_POINT('Ctrl Pts',(-0.332829534430515,-0.978326527256894,
10.3082539354471));
#11422=CARTESIAN_POINT('Ctrl Pts',(0.175201126514412,-1.01615194386632,
10.3322257202373));
#11423=CARTESIAN_POINT('Ctrl Pts',(0.570912684782833,-0.837348131381933,
10.3526616834307));
#11424=CARTESIAN_POINT('Ctrl Pts',(0.812372874444947,-0.581335050023905,
10.3695793154414));
#11425=CARTESIAN_POINT('Ctrl Pts',(0.983676116433903,-0.250820913163252,
10.3874712603802));
#11426=CARTESIAN_POINT('Ctrl Pts',(1.01061901534878,0.226684592654012,10.4097995269886));
#11427=CARTESIAN_POINT('Ctrl Pts',(0.733269268835352,0.72798038254435,10.4365300469703));
#11428=CARTESIAN_POINT('Ctrl Pts',(0.233093165855876,1.00419866522971,10.4631992375404));
#11429=CARTESIAN_POINT('Ctrl Pts',(-0.336165877643461,0.972059073620533,
10.4898068448759));
#11430=CARTESIAN_POINT('Ctrl Pts',(-0.799969685254342,0.642727140263,10.5163536740842));
#11431=CARTESIAN_POINT('Ctrl Pts',(-1.01699704815844,0.118312035325428,
10.5428401065924));
#11432=CARTESIAN_POINT('Ctrl Pts',(-0.92196271867631,-0.439928903735246,
10.5692667693717));
#11433=CARTESIAN_POINT('Ctrl Pts',(-0.545343903600284,-0.86109976629844,
10.5956342393924));
#11434=CARTESIAN_POINT('Ctrl Pts',(-0.00357983942734503,-1.01699776973905,
10.6219431694178));
#11435=CARTESIAN_POINT('Ctrl Pts',(0.536895859987019,-0.861110061278634,
10.6481942447077));
#11436=CARTESIAN_POINT('Ctrl Pts',(0.910778345211294,-0.442480419813451,
10.6743881916688));
#11437=CARTESIAN_POINT('Ctrl Pts',(1.00442833895634,0.109709764210513,10.7005257813949));
#11438=CARTESIAN_POINT('Ctrl Pts',(0.790397648834613,0.625987767469122,
10.7266078184931));
#11439=CARTESIAN_POINT('Ctrl Pts',(0.335451246135889,0.948585082178801,
10.7526351610479));
#11440=CARTESIAN_POINT('Ctrl Pts',(-0.220246780266447,0.979624559336618,
10.7786086842944));
#11441=CARTESIAN_POINT('Ctrl Pts',(-0.706298501153887,0.710807550814349,
10.8045293452089));
#11442=CARTESIAN_POINT('Ctrl Pts',(-0.97430102068363,0.225561067647772,
10.8303980365973));
#11443=CARTESIAN_POINT('Ctrl Pts',(-0.943134026742999,-0.326798203428734,
10.8562159260074));
#11444=CARTESIAN_POINT('Ctrl Pts',(-0.623500527832522,-0.77708962181922,
10.8819836674486));
#11445=CARTESIAN_POINT('Ctrl Pts',(-0.114286877111302,-0.987848109921079,
10.9077031700225));
#11446=CARTESIAN_POINT('Ctrl Pts',(0.427995002062218,-0.89575880106675,
10.9333736290742));
#11447=CARTESIAN_POINT('Ctrl Pts',(0.837323125674483,-0.529580069932072,
10.9590003936702));
#11448=CARTESIAN_POINT('Ctrl Pts',(0.93834816881921,-0.179033497520655,
10.9760482739938));
#11449=CARTESIAN_POINT('Ctrl Pts',(0.938371883484785,-0.00287492837111495,
10.9845738995199));
#11450=CARTESIAN_POINT('Ctrl Pts',(1.0224394592446,0.00362858594397732,
7.80008768273634));
#11451=CARTESIAN_POINT('Ctrl Pts',(1.02241364265261,0.19540078259054,7.80936896800732));
#11452=CARTESIAN_POINT('Ctrl Pts',(0.912365375626032,0.57748816023679,7.82794865742167));
#11453=CARTESIAN_POINT('Ctrl Pts',(0.466303723879016,0.976511784703295,
7.85587267582946));
#11454=CARTESIAN_POINT('Ctrl Pts',(-0.12473483707645,1.07692671916304,7.88385124243725));
#11455=CARTESIAN_POINT('Ctrl Pts',(-0.679785908842397,0.847195663681504,
7.91188381887182));
#11456=CARTESIAN_POINT('Ctrl Pts',(-1.02819315903746,0.356372289452735,
7.9399697564847));
#11457=CARTESIAN_POINT('Ctrl Pts',(-1.06215795437488,-0.245685199795368,
7.96810840972975));
#11458=CARTESIAN_POINT('Ctrl Pts',(-0.770066569818735,-0.774521991341539,
7.99629908755091));
#11459=CARTESIAN_POINT('Ctrl Pts',(-0.240432926725803,-1.06742485611863,
8.0245410726846));
#11460=CARTESIAN_POINT('Ctrl Pts',(0.364933771816083,-1.0335904414025,8.05283360601858));
#11461=CARTESIAN_POINT('Ctrl Pts',(0.860379085372304,-0.682247758833767,
8.08117590069636));
#11462=CARTESIAN_POINT('Ctrl Pts',(1.09335500942013,-0.120192427037716,
8.10956712720536));
#11463=CARTESIAN_POINT('Ctrl Pts',(0.991419462258226,0.480675844038809,
8.13800642480989));
#11464=CARTESIAN_POINT('Ctrl Pts',(0.584737611570177,0.935973198560486,
8.16649288404474));
#11465=CARTESIAN_POINT('Ctrl Pts',(-0.0027678196026674,1.10536381524647,
8.19502559140558));
#11466=CARTESIAN_POINT('Ctrl Pts',(-0.59133830992197,0.935988511200654,
8.22360351453493));
#11467=CARTESIAN_POINT('Ctrl Pts',(-0.984924251409923,0.495548388775854,
8.25116567700538));
#11468=CARTESIAN_POINT('Ctrl Pts',(-1.07847291175567,0.0310816574929332,
8.27345907397737));
#11469=CARTESIAN_POINT('Ctrl Pts',(-1.02459118072371,-0.273105602170713,
8.28833656227911));
#11470=CARTESIAN_POINT('Ctrl Pts',(-0.96248957961835,-0.437297739773922,
8.29684231384406));
#11471=CARTESIAN_POINT('Ctrl Pts',(-0.839511150877903,-0.670321160019251,
8.30960497566622));
#11472=CARTESIAN_POINT('Ctrl Pts',(-0.548303540985154,-0.954553814143627,
8.32876278234068));
#11473=CARTESIAN_POINT('Ctrl Pts',(-0.0248445001511764,-1.10234641140064,
8.35433996388364));
#11474=CARTESIAN_POINT('Ctrl Pts',(0.505244368626293,-0.980683310613957,
8.37994796636545));
#11475=CARTESIAN_POINT('Ctrl Pts',(0.983298938382587,-0.561102157425724,
8.40985911563777));
#11476=CARTESIAN_POINT('Ctrl Pts',(1.15306759627895,0.17600323712225,8.44409052111051));
#11477=CARTESIAN_POINT('Ctrl Pts',(0.773321078747944,0.831505957598933,
8.4783778493315));
#11478=CARTESIAN_POINT('Ctrl Pts',(0.190424898254101,1.09310862502598,8.50842107329988));
#11479=CARTESIAN_POINT('Ctrl Pts',(-0.355521415788955,1.05241611124383,
8.53419886303447));
#11480=CARTESIAN_POINT('Ctrl Pts',(-0.778104439028643,0.779408807091155,
8.55784986417128));
#11481=CARTESIAN_POINT('Ctrl Pts',(-1.01743271691609,0.397361561177328,
8.57936934857403));
#11482=CARTESIAN_POINT('Ctrl Pts',(-1.11987755001356,-0.135106308393046,
8.60521057121674));
#11483=CARTESIAN_POINT('Ctrl Pts',(-0.860210203886423,-0.799841353930079,
8.6375404134144));
#11484=CARTESIAN_POINT('Ctrl Pts',(-0.0861596556698379,-1.17290745782566,
8.67638602671966));
#11485=CARTESIAN_POINT('Ctrl Pts',(0.734967656111525,-0.919467499002295,
8.71527555952678));
#11486=CARTESIAN_POINT('Ctrl Pts',(1.16550630786582,-0.174715119235608,
8.75420591182071));
#11487=CARTESIAN_POINT('Ctrl Pts',(0.973778738558462,0.665697588208069,
8.79317445015984));
#11488=CARTESIAN_POINT('Ctrl Pts',(0.380463090672774,1.06911800335217,8.82567420440926));
#11489=CARTESIAN_POINT('Ctrl Pts',(-0.165164537359199,1.08794158438632,
8.85169301078046));
#11490=CARTESIAN_POINT('Ctrl Pts',(-0.594400866537851,0.938439198965205,
8.87338270538702));
#11491=CARTESIAN_POINT('Ctrl Pts',(-0.95773126151556,0.584213648932498,
8.89725029751952));
#11492=CARTESIAN_POINT('Ctrl Pts',(-1.12103889708631,0.055105611023825,
8.92329682233336));
#11493=CARTESIAN_POINT('Ctrl Pts',(-1.01110710742072,-0.487664602636993,
8.94935728559613));
#11494=CARTESIAN_POINT('Ctrl Pts',(-0.655055427041069,-0.91224848520086,
8.97542181862965));
#11495=CARTESIAN_POINT('Ctrl Pts',(-0.139243614128308,-1.1145127827179,
9.00149832931453));
#11496=CARTESIAN_POINT('Ctrl Pts',(0.36516306280004,-1.05133216304336,9.02540442403775));
#11497=CARTESIAN_POINT('Ctrl Pts',(0.750234379277831,-0.808326308082215,
9.04714316415924));
#11498=CARTESIAN_POINT('Ctrl Pts',(1.07716885680808,-0.36909138500367,9.07323293203551));
#11499=CARTESIAN_POINT('Ctrl Pts',(1.13264226238729,0.348905435514389,9.10585241853449));
#11500=CARTESIAN_POINT('Ctrl Pts',(0.681535489212814,0.912168559624331,
9.13846615527862));
#11501=CARTESIAN_POINT('Ctrl Pts',(0.164491157620536,1.09123311876696,9.1645653126246));
#11502=CARTESIAN_POINT('Ctrl Pts',(-0.313915065303131,1.07428767346862,
9.18740100572472));
#11503=CARTESIAN_POINT('Ctrl Pts',(-0.803557843644582,0.803817864196927,
9.21349549904032));
#11504=CARTESIAN_POINT('Ctrl Pts',(-1.10777522245362,0.253279572730345,
9.24284916045016));
#11505=CARTESIAN_POINT('Ctrl Pts',(-1.07262556922497,-0.375096829106732,
9.27219864048019));
#11506=CARTESIAN_POINT('Ctrl Pts',(-0.775849519172851,-0.792323064162487,
9.29610586960291));
#11507=CARTESIAN_POINT('Ctrl Pts',(-0.371328745506812,-1.03953633075296,
9.31892645589477));
#11508=CARTESIAN_POINT('Ctrl Pts',(0.0376304846545741,-1.11184105971114,
9.33848334826187));
#11509=CARTESIAN_POINT('Ctrl Pts',(0.477752265059943,-0.993378524589055,
9.36020520881827));
#11510=CARTESIAN_POINT('Ctrl Pts',(0.807452663693637,-0.750309094977912,
9.37975248696025));
#11511=CARTESIAN_POINT('Ctrl Pts',(1.02542831143796,-0.403287461382024,
9.3992915884546));
#11512=CARTESIAN_POINT('Ctrl Pts',(1.09520570424478,-0.0343996015918939,
9.41719819112087));
#11513=CARTESIAN_POINT('Ctrl Pts',(1.04766435799285,0.300821003164569,9.4334730419063));
#11514=CARTESIAN_POINT('Ctrl Pts',(0.882134941333648,0.671933761076852,
9.4529986725804));
#11515=CARTESIAN_POINT('Ctrl Pts',(0.492704809338165,1.0203555390095,9.4773907315634));
#11516=CARTESIAN_POINT('Ctrl Pts',(-0.125813239292152,1.12538522726572,
9.50664807519627));
#11517=CARTESIAN_POINT('Ctrl Pts',(-0.607916474994097,0.925314738520527,
9.5310110810177));
#11518=CARTESIAN_POINT('Ctrl Pts',(-0.886009132880398,0.630281874283733,
9.55049558512337));
#11519=CARTESIAN_POINT('Ctrl Pts',(-1.07254869382692,0.270488248614126,
9.56997311484588));
#11520=CARTESIAN_POINT('Ctrl Pts',(-1.10201013131539,-0.25001327256632,
9.59430238061315));
#11521=CARTESIAN_POINT('Ctrl Pts',(-0.799358428997046,-0.797323059937847,
9.62347692829483));
#11522=CARTESIAN_POINT('Ctrl Pts',(-0.252578030159201,-1.09942897214462,
9.65262644221176));
#11523=CARTESIAN_POINT('Ctrl Pts',(0.370672782655161,-1.06436218073861,
9.68175071510106));
#11524=CARTESIAN_POINT('Ctrl Pts',(0.879222485658297,-0.703403547720322,
9.71084774442572));
#11525=CARTESIAN_POINT('Ctrl Pts',(1.11755902291746,-0.12776947340514,9.73991636014012));
#11526=CARTESIAN_POINT('Ctrl Pts',(1.01322037204631,0.485811010865536,9.76895508611072));
#11527=CARTESIAN_POINT('Ctrl Pts',(0.598843742169754,0.949332890885439,
9.79796253896268));
#11528=CARTESIAN_POINT('Ctrl Pts',(0.00212031341932294,1.12116294453614,
9.82693748941955));
#11529=CARTESIAN_POINT('Ctrl Pts',(-0.594030577562524,0.949371974584455,
9.85587828377846));
#11530=CARTESIAN_POINT('Ctrl Pts',(-0.991227126988807,0.504456962371331,
9.88371366780931));
#11531=CARTESIAN_POINT('Ctrl Pts',(-1.10366008874695,-0.0526856529500433,
9.91044589924098));
#11532=CARTESIAN_POINT('Ctrl Pts',(-0.942838790043787,-0.573096610903901,
9.93608238452499));
#11533=CARTESIAN_POINT('Ctrl Pts',(-0.585724594591535,-0.921582228722216,
9.95955452943091));
#11534=CARTESIAN_POINT('Ctrl Pts',(-0.163975590932816,-1.06829755406478,
9.98086822993116));
#11535=CARTESIAN_POINT('Ctrl Pts',(0.372168170774437,-1.04971711604162,
10.0064236491231));
#11536=CARTESIAN_POINT('Ctrl Pts',(0.837477772259037,-0.733785381710125,
10.0319384111643));
#11537=CARTESIAN_POINT('Ctrl Pts',(1.049292306327,-0.242423951232681,10.0574181798459));
#11538=CARTESIAN_POINT('Ctrl Pts',(1.0710034914769,0.29080545818794,10.0828736616323));
#11539=CARTESIAN_POINT('Ctrl Pts',(0.72099131572971,0.89885340658251,10.1146376758435));
#11540=CARTESIAN_POINT('Ctrl Pts',(-0.0838294263341789,1.14666175739243,
10.1526781887287));
#11541=CARTESIAN_POINT('Ctrl Pts',(-0.753997956341837,0.822259906126611,
10.1864162007806));
#11542=CARTESIAN_POINT('Ctrl Pts',(-1.05275079101018,0.270909471727262,
10.2158844277476));
#11543=CARTESIAN_POINT('Ctrl Pts',(-1.05256683050461,-0.26474101391336,
10.2411067512839));
#11544=CARTESIAN_POINT('Ctrl Pts',(-0.796701237850394,-0.735095856462346,
10.2662893641572));
#11545=CARTESIAN_POINT('Ctrl Pts',(-0.34759897431464,-1.02472783459927,
10.2914312125966));
#11546=CARTESIAN_POINT('Ctrl Pts',(0.18447326483658,-1.06437052854044,10.3165357251281));
#11547=CARTESIAN_POINT('Ctrl Pts',(0.599067458247316,-0.877055322325079,
10.3379407915222));
#11548=CARTESIAN_POINT('Ctrl Pts',(0.852159422370925,-0.608714393671463,
10.3556713883906));
#11549=CARTESIAN_POINT('Ctrl Pts',(1.03175866217658,-0.262202962400976,
10.3744275198819));
#11550=CARTESIAN_POINT('Ctrl Pts',(1.06003703932392,0.238542818252046,10.3978364643517));
#11551=CARTESIAN_POINT('Ctrl Pts',(0.769079304176225,0.764498896052599,
10.4258758659065));
#11552=CARTESIAN_POINT('Ctrl Pts',(0.244120099803413,1.05442656731387,10.4538609075553));
#11553=CARTESIAN_POINT('Ctrl Pts',(-0.353571270507426,1.02070521861313,
10.4817919929746));
#11554=CARTESIAN_POINT('Ctrl Pts',(-0.840707898088968,0.67483086915919,
10.5096681144061));
#11555=CARTESIAN_POINT('Ctrl Pts',(-1.06872999263526,0.123899612590722,
10.5374889758409));
#11556=CARTESIAN_POINT('Ctrl Pts',(-0.968881292507578,-0.462723739670875,
10.5652540330952));
#11557=CARTESIAN_POINT('Ctrl Pts',(-0.573043307192763,-0.905408458289749,
10.5929629214798));
#11558=CARTESIAN_POINT('Ctrl Pts',(-0.00352082082609249,-1.06930551127307,
10.6206152641652));
#11559=CARTESIAN_POINT('Ctrl Pts',(0.564731071947371,-0.90541400189164,
10.6482107513056));
#11560=CARTESIAN_POINT('Ctrl Pts',(0.957869636830534,-0.465229288689372,
10.675749107199));
#11561=CARTESIAN_POINT('Ctrl Pts',(1.05634881760394,0.115433979910032,10.7032301036035));
#11562=CARTESIAN_POINT('Ctrl Pts',(0.83127262512651,0.658347260291639,10.7306535506042));
#11563=CARTESIAN_POINT('Ctrl Pts',(0.352855070853646,0.997579943766369,
10.7580193078072));
#11564=CARTESIAN_POINT('Ctrl Pts',(-0.231480179248419,1.03021016071997,
10.7853272583561));
#11565=CARTESIAN_POINT('Ctrl Pts',(-0.742529937572376,0.747555014282395,
10.8125773674657));
#11566=CARTESIAN_POINT('Ctrl Pts',(-1.02427277250167,0.237405701771815,
10.8397695463441));
#11567=CARTESIAN_POINT('Ctrl Pts',(-0.991498148688415,-0.343196952014676,
10.8669039522539));
#11568=CARTESIAN_POINT('Ctrl Pts',(-0.655579551142097,-0.81640152144281,
10.8939803118662));
#11569=CARTESIAN_POINT('Ctrl Pts',(-0.120565700495315,-1.03781837274451,
10.9209994211754));
#11570=CARTESIAN_POINT('Ctrl Pts',(0.44900506988111,-0.941049432983352,
10.9479597810765));
#11571=CARTESIAN_POINT('Ctrl Pts',(0.878779001046494,-0.556545520129311,
10.9748651152608));
#11572=CARTESIAN_POINT('Ctrl Pts',(0.984764947260803,-0.188518733496692,
10.9927592993211));
#11573=CARTESIAN_POINT('Ctrl Pts',(0.984789826393123,-0.00371020912213119,
11.0017035606219));
#11574=CARTESIAN_POINT('Ctrl Pts',(0.999999511922295,0.00362556505265694,
7.80008768273634));
#11575=CARTESIAN_POINT('Ctrl Pts',(0.999974254701651,0.191242609375982,
7.80916786923111));
#11576=CARTESIAN_POINT('Ctrl Pts',(0.892341067491657,0.564938782877452,
7.82733932423682));
#11577=CARTESIAN_POINT('Ctrl Pts',(0.456009237357814,0.955278731473674,
7.85465504855182));
#11578=CARTESIAN_POINT('Ctrl Pts',(-0.122182810478375,1.05350592491678,
7.88202502929242));
#11579=CARTESIAN_POINT('Ctrl Pts',(-0.665220911419956,0.828753483606749,
7.90945086692426));
#11580=CARTESIAN_POINT('Ctrl Pts',(-1.00612665101876,0.348504727673495,
7.93693161942117));
#11581=CARTESIAN_POINT('Ctrl Pts',(-1.03937057711115,-0.24065277058934,
7.96446742990799));
#11582=CARTESIAN_POINT('Ctrl Pts',(-0.753506480379588,-0.758233234780652,
7.99205790686499));
#11583=CARTESIAN_POINT('Ctrl Pts',(-0.23507859765888,-1.04495072049649,
8.01970284677932));
#11584=CARTESIAN_POINT('Ctrl Pts',(0.357583215672993,-1.01183827364816,
8.04740190675199));
#11585=CARTESIAN_POINT('Ctrl Pts',(0.842723866190013,-0.667819008067397,
8.07515475263842));
#11586=CARTESIAN_POINT('Ctrl Pts',(1.07090748459127,-0.117361728527591,
8.1029609908626));
#11587=CARTESIAN_POINT('Ctrl Pts',(0.971068313490196,0.471237645030074,
8.13082019638131));
#11588=CARTESIAN_POINT('Ctrl Pts',(0.572615291983895,0.917345600069376,
8.15873190469605));
#11589=CARTESIAN_POINT('Ctrl Pts',(-0.00315068596155565,1.08336827030711,
8.18669561143439));
#11590=CARTESIAN_POINT('Ctrl Pts',(-0.580114085036881,0.917350780124834,
8.21471077684478));
#11591=CARTESIAN_POINT('Ctrl Pts',(-0.966051395769627,0.48549839913134,
8.24173733490367));
#11592=CARTESIAN_POINT('Ctrl Pts',(-1.05781582749726,0.0299567596628159,
8.2636033984339));
#11593=CARTESIAN_POINT('Ctrl Pts',(-1.00496213983024,-0.268439331682945,
8.27819794787177));
#11594=CARTESIAN_POINT('Ctrl Pts',(-0.94403781713285,-0.429519542479439,
8.28654256698954));
#11595=CARTESIAN_POINT('Ctrl Pts',(-0.823382078993268,-0.658140969899007,
8.29906435736913));
#11596=CARTESIAN_POINT('Ctrl Pts',(-0.537625296367964,-0.93706913925231,
8.31786521711992));
#11597=CARTESIAN_POINT('Ctrl Pts',(-0.0238288726443125,-1.08214769701979,
8.34297130007593));
#11598=CARTESIAN_POINT('Ctrl Pts',(0.496636287796273,-0.96271505408145,
8.36811512451513));
#11599=CARTESIAN_POINT('Ctrl Pts',(0.966152438091784,-0.550650417462692,
8.39749297986939));
#11600=CARTESIAN_POINT('Ctrl Pts',(1.13301488484768,0.17354695961988,8.43112871623582));
#11601=CARTESIAN_POINT('Ctrl Pts',(0.759782029367692,0.81792928250629,8.46483592073065));
#11602=CARTESIAN_POINT('Ctrl Pts',(0.18659690053678,1.07520238454981,8.49438045894607));
#11603=CARTESIAN_POINT('Ctrl Pts',(-0.350443601960556,1.03519669411318,
8.51973848476555));
#11604=CARTESIAN_POINT('Ctrl Pts',(-0.766297161890012,0.766560498033478,
8.54301401492018));
#11605=CARTESIAN_POINT('Ctrl Pts',(-1.00188555557132,0.390501874334262,
8.56419748306598));
#11606=CARTESIAN_POINT('Ctrl Pts',(-1.10276576842174,-0.133757727725488,
8.5896418232172));
#11607=CARTESIAN_POINT('Ctrl Pts',(-0.847050948528023,-0.7885712029239,
8.6214918164511));
#11608=CARTESIAN_POINT('Ctrl Pts',(-0.0842079511184448,-1.15633714773807,
8.65978061793639));
#11609=CARTESIAN_POINT('Ctrl Pts',(0.72557322963091,-0.906499072035091,
8.69813561803015));
#11610=CARTESIAN_POINT('Ctrl Pts',(1.15047751535783,-0.171671665185466,
8.73655413319947));
#11611=CARTESIAN_POINT('Ctrl Pts',(0.961273159473049,0.658124915791643,
8.77503338584849));
#11612=CARTESIAN_POINT('Ctrl Pts',(0.375126711265494,1.05675920723847,8.80714766479813));
#11613=CARTESIAN_POINT('Ctrl Pts',(-0.164183045710825,1.07538023554299,
8.8328665668906));
#11614=CARTESIAN_POINT('Ctrl Pts',(-0.588587403918608,0.927569264768944,
8.85431383603483));
#11615=CARTESIAN_POINT('Ctrl Pts',(-0.947989492545562,0.577208917394653,
8.87792434906622));
#11616=CARTESIAN_POINT('Ctrl Pts',(-1.10961450093061,0.0536146968196933,
8.90370345540594));
#11617=CARTESIAN_POINT('Ctrl Pts',(-1.00082022593385,-0.483727092204472,
8.92950382341385));
#11618=CARTESIAN_POINT('Ctrl Pts',(-0.648169490504554,-0.904286310022195,
8.95532452406706));
#11619=CARTESIAN_POINT('Ctrl Pts',(-0.137073525470092,-1.1047399934849,
8.98116461266558));
#11620=CARTESIAN_POINT('Ctrl Pts',(0.362995552358674,-1.04213062048012,
9.0048682588092));
#11621=CARTESIAN_POINT('Ctrl Pts',(0.744903368537152,-0.801138176501351,
9.02642976126975));
#11622=CARTESIAN_POINT('Ctrl Pts',(1.06927029269131,-0.365389501861442,
9.05231612054031));
#11623=CARTESIAN_POINT('Ctrl Pts',(1.12442623960627,0.347295239484755,9.08469656290588));
#11624=CARTESIAN_POINT('Ctrl Pts',(0.676375081319218,0.906916376424927,
9.11710422215215));
#11625=CARTESIAN_POINT('Ctrl Pts',(0.162505682592346,1.08489901523682,9.14304497362832));
#11626=CARTESIAN_POINT('Ctrl Pts',(-0.313134592199748,1.06806757295122,
9.16575116654966));
#11627=CARTESIAN_POINT('Ctrl Pts',(-0.80020652042605,0.79906113083438,9.19171186155256));
#11628=CARTESIAN_POINT('Ctrl Pts',(-1.1030130064212,0.251155630516143,9.22093071361268));
#11629=CARTESIAN_POINT('Ctrl Pts',(-1.06806000491819,-0.374587327913118,
9.25016115867103));
#11630=CARTESIAN_POINT('Ctrl Pts',(-0.772382685892504,-0.790331103336901,
9.27398680631869));
#11631=CARTESIAN_POINT('Ctrl Pts',(-0.369190625906315,-1.03674084848642,
9.29673431868371));
#11632=CARTESIAN_POINT('Ctrl Pts',(0.038576143908095,-1.10885924555696,
9.31623572825941));
#11633=CARTESIAN_POINT('Ctrl Pts',(0.477637122556786,-0.990697811322314,
9.33790778885712));
#11634=CARTESIAN_POINT('Ctrl Pts',(0.806650901305872,-0.74814670656117,
9.35741515109002));
#11635=CARTESIAN_POINT('Ctrl Pts',(1.02427838601106,-0.401712335365787,
9.37692457700679));
#11636=CARTESIAN_POINT('Ctrl Pts',(1.0939769734331,-0.0333100781542004,
9.39480970049716));
#11637=CARTESIAN_POINT('Ctrl Pts',(1.04649131988823,0.301575311206996,9.4110697587252));
#11638=CARTESIAN_POINT('Ctrl Pts',(0.881091959620118,0.67241835967004,9.43058245602211));
#11639=CARTESIAN_POINT('Ctrl Pts',(0.491781434765328,1.02078793932956,9.45497403322699));
#11640=CARTESIAN_POINT('Ctrl Pts',(-0.12690622562046,1.12590240218231,9.48424354952418));
#11641=CARTESIAN_POINT('Ctrl Pts',(-0.609455917268022,0.925702271760676,
9.50863324396813));
#11642=CARTESIAN_POINT('Ctrl Pts',(-0.887901221690915,0.630308788370616,
9.52814330365954));
#11643=CARTESIAN_POINT('Ctrl Pts',(-1.07473168029324,0.269973249594665,
9.54765198252425));
#11644=CARTESIAN_POINT('Ctrl Pts',(-1.10429179277937,-0.251571030257534,
9.57203477138778));
#11645=CARTESIAN_POINT('Ctrl Pts',(-0.800909981683876,-0.800300061810875,
9.60128772802457));
#11646=CARTESIAN_POINT('Ctrl Pts',(-0.252449360054481,-1.10339503360944,
9.63053279474191));
#11647=CARTESIAN_POINT('Ctrl Pts',(0.373097965965379,-1.06824993186655,
9.65976848374119));
#11648=CARTESIAN_POINT('Ctrl Pts',(0.883833752107615,-0.705802685092957,
9.68899331286683));
#11649=CARTESIAN_POINT('Ctrl Pts',(1.12336062251109,-0.127424704798401,
9.71820580950298));
#11650=CARTESIAN_POINT('Ctrl Pts',(1.01851100341375,0.489451283507362,9.7474045069875));
#11651=CARTESIAN_POINT('Ctrl Pts',(0.601719134479875,0.955745657723928,
9.7765879476835));
#11652=CARTESIAN_POINT('Ctrl Pts',(0.00114764771726767,1.12873118183179,
9.80575469579441));
#11653=CARTESIAN_POINT('Ctrl Pts',(-0.599201162150444,0.955775323307818,
9.83490331154648));
#11654=CARTESIAN_POINT('Ctrl Pts',(-0.999441525170258,0.507519999720283,
9.86295352909998));
#11655=CARTESIAN_POINT('Ctrl Pts',(-1.11281367201976,-0.0541281101275826,
9.88990656850941));
#11656=CARTESIAN_POINT('Ctrl Pts',(-0.950656776962806,-0.578991698652294,
9.91576396161208));
#11657=CARTESIAN_POINT('Ctrl Pts',(-0.590339529048702,-0.930637197709755,
9.93944961788225));
#11658=CARTESIAN_POINT('Ctrl Pts',(-0.164606104863989,-1.07875415066616,
9.96096785470298));
#11659=CARTESIAN_POINT('Ctrl Pts',(0.376774813272184,-1.06001813820014,
9.98677462212391));
#11660=CARTESIAN_POINT('Ctrl Pts',(0.846936223245377,-0.740877146125449,
10.0125579187175));
#11661=CARTESIAN_POINT('Ctrl Pts',(1.06107082068352,-0.244205647020787,
10.0383162020965));
#11662=CARTESIAN_POINT('Ctrl Pts',(1.08304241869915,0.294959566025181,10.0640572896683));
#11663=CARTESIAN_POINT('Ctrl Pts',(0.729014765427379,0.91016891175548,10.0962004771028));
#11664=CARTESIAN_POINT('Ctrl Pts',(-0.0857101331349617,1.16113591721249,
10.1347162317012));
#11665=CARTESIAN_POINT('Ctrl Pts',(-0.764643776951617,0.832591967114145,
10.1689000478027));
#11666=CARTESIAN_POINT('Ctrl Pts',(-1.0674640769428,0.273793097090764,10.1987708394967));
#11667=CARTESIAN_POINT('Ctrl Pts',(-1.06731019456222,-0.269314357950732,
10.22434609796));
#11668=CARTESIAN_POINT('Ctrl Pts',(-0.807788715964582,-0.746430097707613,
10.2498922819076));
#11669=CARTESIAN_POINT('Ctrl Pts',(-0.352065023972404,-1.04036411773073,
10.275408603128));
#11670=CARTESIAN_POINT('Ctrl Pts',(0.18806187608402,-1.08063605589285,10.3008942987819));
#11671=CARTESIAN_POINT('Ctrl Pts',(0.609132779330515,-0.890423751871434,
10.3226365334534));
#11672=CARTESIAN_POINT('Ctrl Pts',(0.866237924373777,-0.61783839929423,
10.3406489137734));
#11673=CARTESIAN_POINT('Ctrl Pts',(1.04872505851243,-0.26577216648544,10.3597071335657));
#11674=CARTESIAN_POINT('Ctrl Pts',(1.07750116603121,0.243190015038482,10.3835038803323));
#11675=CARTESIAN_POINT('Ctrl Pts',(0.781688530878207,0.777999980609408,
10.4120173608425));
#11676=CARTESIAN_POINT('Ctrl Pts',(0.247719136142376,1.07295015546241,10.4404872688827));
#11677=CARTESIAN_POINT('Ctrl Pts',(-0.360486616831365,1.03867188015668,
10.4689126947258));
#11678=CARTESIAN_POINT('Ctrl Pts',(-0.856395421979649,0.686612064758622,
10.4972927514314));
#11679=CARTESIAN_POINT('Ctrl Pts',(-1.08862861454113,0.125592182065228,
10.5256265935356));
#11680=CARTESIAN_POINT('Ctrl Pts',(-0.986944606168628,-0.472001059894419,
10.5539134034074));
#11681=CARTESIAN_POINT('Ctrl Pts',(-0.583594151562567,-0.923132799570535,
10.5821523997639));
#11682=CARTESIAN_POINT('Ctrl Pts',(-0.00304950196324622,-1.09023227406354,
10.6103428416619));
#11683=CARTESIAN_POINT('Ctrl Pts',(0.576397100829433,-0.923141572582211,
10.6384840153271));
#11684=CARTESIAN_POINT('Ctrl Pts',(0.977415745977647,-0.474174920735025,
10.666575250779));
#11685=CARTESIAN_POINT('Ctrl Pts',(1.07791854333959,0.118262177227866,10.6946159100158));
#11686=CARTESIAN_POINT('Ctrl Pts',(0.848237687346995,0.672348815808936,
10.7226053954193));
#11687=CARTESIAN_POINT('Ctrl Pts',(0.35987034323251,1.01866632704243,10.750543145368));
#11688=CARTESIAN_POINT('Ctrl Pts',(-0.23677931351889,1.05200727853759,10.7784286311663));
#11689=CARTESIAN_POINT('Ctrl Pts',(-0.758730842080508,0.763346883548158,
10.8062613781485));
#11690=CARTESIAN_POINT('Ctrl Pts',(-1.04655744183574,0.242222537004657,
10.8340409125563));
#11691=CARTESIAN_POINT('Ctrl Pts',(-1.01308793288556,-0.351003613269005,
10.8617668734456));
#11692=CARTESIAN_POINT('Ctrl Pts',(-0.669814425530371,-0.834593746223134,
10.889438771651));
#11693=CARTESIAN_POINT('Ctrl Pts',(-0.122977155730889,-1.06092281666227,
10.9170565165848));
#11694=CARTESIAN_POINT('Ctrl Pts',(0.459284142389985,-0.962004532278344,
10.9446192376113));
#11695=CARTESIAN_POINT('Ctrl Pts',(0.898703292351648,-0.568910379520766,
10.9721279252064));
#11696=CARTESIAN_POINT('Ctrl Pts',(1.0071027576084,-0.192548907318078,10.9904290025552));
#11697=CARTESIAN_POINT('Ctrl Pts',(1.00712819276269,-0.00361011030918905,
10.999573158519));
#11698=CARTESIAN_POINT('',(0.999999511922295,0.00362556505265694,7.80008768273634));
#11699=CARTESIAN_POINT('Origin',(1.,0.,7.875));
#11700=CARTESIAN_POINT('',(1.00712819276269,-0.00361011030918906,10.999573158519));
#11701=CARTESIAN_POINT('Ctrl Pts',(0.999999511922295,0.00362556505265694,
7.80008768273634));
#11702=CARTESIAN_POINT('Ctrl Pts',(0.999974254701651,0.191242609375982,
7.80916786923111));
#11703=CARTESIAN_POINT('Ctrl Pts',(0.892341067491657,0.564938782877452,
7.82733932423682));
#11704=CARTESIAN_POINT('Ctrl Pts',(0.456009237357814,0.955278731473674,
7.85465504855182));
#11705=CARTESIAN_POINT('Ctrl Pts',(-0.122182810478375,1.05350592491678,
7.88202502929242));
#11706=CARTESIAN_POINT('Ctrl Pts',(-0.665220911419956,0.828753483606749,
7.90945086692426));
#11707=CARTESIAN_POINT('Ctrl Pts',(-1.00612665101876,0.348504727673495,
7.93693161942117));
#11708=CARTESIAN_POINT('Ctrl Pts',(-1.03937057711115,-0.24065277058934,
7.96446742990799));
#11709=CARTESIAN_POINT('Ctrl Pts',(-0.753506480379588,-0.758233234780652,
7.99205790686499));
#11710=CARTESIAN_POINT('Ctrl Pts',(-0.23507859765888,-1.04495072049649,
8.01970284677932));
#11711=CARTESIAN_POINT('Ctrl Pts',(0.357583215672993,-1.01183827364816,
8.04740190675199));
#11712=CARTESIAN_POINT('Ctrl Pts',(0.842723866190013,-0.667819008067397,
8.07515475263842));
#11713=CARTESIAN_POINT('Ctrl Pts',(1.07090748459127,-0.117361728527591,
8.1029609908626));
#11714=CARTESIAN_POINT('Ctrl Pts',(0.971068313490196,0.471237645030074,
8.13082019638131));
#11715=CARTESIAN_POINT('Ctrl Pts',(0.572615291983895,0.917345600069376,
8.15873190469605));
#11716=CARTESIAN_POINT('Ctrl Pts',(-0.00315068596155565,1.08336827030711,
8.18669561143439));
#11717=CARTESIAN_POINT('Ctrl Pts',(-0.580114085036881,0.917350780124834,
8.21471077684478));
#11718=CARTESIAN_POINT('Ctrl Pts',(-0.966051395769627,0.48549839913134,
8.24173733490367));
#11719=CARTESIAN_POINT('Ctrl Pts',(-1.05781582749726,0.0299567596628159,
8.2636033984339));
#11720=CARTESIAN_POINT('Ctrl Pts',(-1.00496213983024,-0.268439331682945,
8.27819794787177));
#11721=CARTESIAN_POINT('Ctrl Pts',(-0.94403781713285,-0.429519542479439,
8.28654256698954));
#11722=CARTESIAN_POINT('Ctrl Pts',(-0.823382078993268,-0.658140969899007,
8.29906435736913));
#11723=CARTESIAN_POINT('Ctrl Pts',(-0.537625296367964,-0.93706913925231,
8.31786521711992));
#11724=CARTESIAN_POINT('Ctrl Pts',(-0.0238288726443125,-1.08214769701979,
8.34297130007593));
#11725=CARTESIAN_POINT('Ctrl Pts',(0.496636287796273,-0.96271505408145,
8.36811512451513));
#11726=CARTESIAN_POINT('Ctrl Pts',(0.966152438091784,-0.550650417462692,
8.39749297986939));
#11727=CARTESIAN_POINT('Ctrl Pts',(1.13301488484768,0.17354695961988,8.43112871623582));
#11728=CARTESIAN_POINT('Ctrl Pts',(0.759782029367692,0.81792928250629,8.46483592073065));
#11729=CARTESIAN_POINT('Ctrl Pts',(0.18659690053678,1.07520238454981,8.49438045894607));
#11730=CARTESIAN_POINT('Ctrl Pts',(-0.350443601960556,1.03519669411318,
8.51973848476555));
#11731=CARTESIAN_POINT('Ctrl Pts',(-0.766297161890012,0.766560498033478,
8.54301401492018));
#11732=CARTESIAN_POINT('Ctrl Pts',(-1.00188555557132,0.390501874334262,
8.56419748306598));
#11733=CARTESIAN_POINT('Ctrl Pts',(-1.10276576842174,-0.133757727725488,
8.5896418232172));
#11734=CARTESIAN_POINT('Ctrl Pts',(-0.847050948528023,-0.7885712029239,
8.6214918164511));
#11735=CARTESIAN_POINT('Ctrl Pts',(-0.0842079511184448,-1.15633714773807,
8.65978061793639));
#11736=CARTESIAN_POINT('Ctrl Pts',(0.72557322963091,-0.906499072035091,
8.69813561803015));
#11737=CARTESIAN_POINT('Ctrl Pts',(1.15047751535783,-0.171671665185466,
8.73655413319947));
#11738=CARTESIAN_POINT('Ctrl Pts',(0.961273159473049,0.658124915791643,
8.77503338584849));
#11739=CARTESIAN_POINT('Ctrl Pts',(0.375126711265494,1.05675920723847,8.80714766479813));
#11740=CARTESIAN_POINT('Ctrl Pts',(-0.164183045710825,1.07538023554299,
8.8328665668906));
#11741=CARTESIAN_POINT('Ctrl Pts',(-0.588587403918608,0.927569264768944,
8.85431383603483));
#11742=CARTESIAN_POINT('Ctrl Pts',(-0.947989492545562,0.577208917394653,
8.87792434906622));
#11743=CARTESIAN_POINT('Ctrl Pts',(-1.10961450093061,0.0536146968196933,
8.90370345540594));
#11744=CARTESIAN_POINT('Ctrl Pts',(-1.00082022593385,-0.483727092204472,
8.92950382341385));
#11745=CARTESIAN_POINT('Ctrl Pts',(-0.648169490504554,-0.904286310022195,
8.95532452406706));
#11746=CARTESIAN_POINT('Ctrl Pts',(-0.137073525470092,-1.1047399934849,
8.98116461266558));
#11747=CARTESIAN_POINT('Ctrl Pts',(0.362995552358674,-1.04213062048012,
9.0048682588092));
#11748=CARTESIAN_POINT('Ctrl Pts',(0.744903368537152,-0.801138176501351,
9.02642976126975));
#11749=CARTESIAN_POINT('Ctrl Pts',(1.06927029269131,-0.365389501861442,
9.05231612054031));
#11750=CARTESIAN_POINT('Ctrl Pts',(1.12442623960627,0.347295239484755,9.08469656290588));
#11751=CARTESIAN_POINT('Ctrl Pts',(0.676375081319218,0.906916376424927,
9.11710422215215));
#11752=CARTESIAN_POINT('Ctrl Pts',(0.162505682592346,1.08489901523682,9.14304497362832));
#11753=CARTESIAN_POINT('Ctrl Pts',(-0.313134592199748,1.06806757295122,
9.16575116654966));
#11754=CARTESIAN_POINT('Ctrl Pts',(-0.80020652042605,0.79906113083438,9.19171186155256));
#11755=CARTESIAN_POINT('Ctrl Pts',(-1.1030130064212,0.251155630516143,9.22093071361268));
#11756=CARTESIAN_POINT('Ctrl Pts',(-1.06806000491819,-0.374587327913118,
9.25016115867103));
#11757=CARTESIAN_POINT('Ctrl Pts',(-0.772382685892504,-0.790331103336901,
9.27398680631869));
#11758=CARTESIAN_POINT('Ctrl Pts',(-0.369190625906315,-1.03674084848642,
9.29673431868371));
#11759=CARTESIAN_POINT('Ctrl Pts',(0.038576143908095,-1.10885924555696,
9.31623572825941));
#11760=CARTESIAN_POINT('Ctrl Pts',(0.477637122556786,-0.990697811322314,
9.33790778885712));
#11761=CARTESIAN_POINT('Ctrl Pts',(0.806650901305872,-0.74814670656117,
9.35741515109002));
#11762=CARTESIAN_POINT('Ctrl Pts',(1.02427838601106,-0.401712335365787,
9.37692457700679));
#11763=CARTESIAN_POINT('Ctrl Pts',(1.0939769734331,-0.0333100781542004,
9.39480970049716));
#11764=CARTESIAN_POINT('Ctrl Pts',(1.04649131988823,0.301575311206996,9.4110697587252));
#11765=CARTESIAN_POINT('Ctrl Pts',(0.881091959620118,0.67241835967004,9.43058245602211));
#11766=CARTESIAN_POINT('Ctrl Pts',(0.491781434765328,1.02078793932956,9.45497403322699));
#11767=CARTESIAN_POINT('Ctrl Pts',(-0.12690622562046,1.12590240218231,9.48424354952418));
#11768=CARTESIAN_POINT('Ctrl Pts',(-0.609455917268022,0.925702271760676,
9.50863324396813));
#11769=CARTESIAN_POINT('Ctrl Pts',(-0.887901221690915,0.630308788370616,
9.52814330365954));
#11770=CARTESIAN_POINT('Ctrl Pts',(-1.07473168029324,0.269973249594665,
9.54765198252425));
#11771=CARTESIAN_POINT('Ctrl Pts',(-1.10429179277937,-0.251571030257534,
9.57203477138778));
#11772=CARTESIAN_POINT('Ctrl Pts',(-0.800909981683876,-0.800300061810875,
9.60128772802457));
#11773=CARTESIAN_POINT('Ctrl Pts',(-0.252449360054481,-1.10339503360944,
9.63053279474191));
#11774=CARTESIAN_POINT('Ctrl Pts',(0.373097965965379,-1.06824993186655,
9.65976848374119));
#11775=CARTESIAN_POINT('Ctrl Pts',(0.883833752107615,-0.705802685092957,
9.68899331286683));
#11776=CARTESIAN_POINT('Ctrl Pts',(1.12336062251109,-0.127424704798401,
9.71820580950298));
#11777=CARTESIAN_POINT('Ctrl Pts',(1.01851100341375,0.489451283507362,9.7474045069875));
#11778=CARTESIAN_POINT('Ctrl Pts',(0.601719134479875,0.955745657723928,
9.7765879476835));
#11779=CARTESIAN_POINT('Ctrl Pts',(0.00114764771726767,1.12873118183179,
9.80575469579441));
#11780=CARTESIAN_POINT('Ctrl Pts',(-0.599201162150444,0.955775323307818,
9.83490331154648));
#11781=CARTESIAN_POINT('Ctrl Pts',(-0.999441525170258,0.507519999720283,
9.86295352909998));
#11782=CARTESIAN_POINT('Ctrl Pts',(-1.11281367201976,-0.0541281101275826,
9.88990656850941));
#11783=CARTESIAN_POINT('Ctrl Pts',(-0.950656776962806,-0.578991698652294,
9.91576396161208));
#11784=CARTESIAN_POINT('Ctrl Pts',(-0.590339529048702,-0.930637197709755,
9.93944961788225));
#11785=CARTESIAN_POINT('Ctrl Pts',(-0.164606104863989,-1.07875415066616,
9.96096785470298));
#11786=CARTESIAN_POINT('Ctrl Pts',(0.376774813272184,-1.06001813820014,
9.98677462212391));
#11787=CARTESIAN_POINT('Ctrl Pts',(0.846936223245377,-0.740877146125449,
10.0125579187175));
#11788=CARTESIAN_POINT('Ctrl Pts',(1.06107082068352,-0.244205647020787,
10.0383162020965));
#11789=CARTESIAN_POINT('Ctrl Pts',(1.08304241869915,0.294959566025181,10.0640572896683));
#11790=CARTESIAN_POINT('Ctrl Pts',(0.729014765427379,0.91016891175548,10.0962004771028));
#11791=CARTESIAN_POINT('Ctrl Pts',(-0.0857101331349617,1.16113591721249,
10.1347162317012));
#11792=CARTESIAN_POINT('Ctrl Pts',(-0.764643776951617,0.832591967114145,
10.1689000478027));
#11793=CARTESIAN_POINT('Ctrl Pts',(-1.0674640769428,0.273793097090764,10.1987708394967));
#11794=CARTESIAN_POINT('Ctrl Pts',(-1.06731019456222,-0.269314357950732,
10.22434609796));
#11795=CARTESIAN_POINT('Ctrl Pts',(-0.807788715964582,-0.746430097707613,
10.2498922819076));
#11796=CARTESIAN_POINT('Ctrl Pts',(-0.352065023972404,-1.04036411773073,
10.275408603128));
#11797=CARTESIAN_POINT('Ctrl Pts',(0.18806187608402,-1.08063605589285,10.3008942987819));
#11798=CARTESIAN_POINT('Ctrl Pts',(0.609132779330515,-0.890423751871434,
10.3226365334534));
#11799=CARTESIAN_POINT('Ctrl Pts',(0.866237924373777,-0.61783839929423,
10.3406489137734));
#11800=CARTESIAN_POINT('Ctrl Pts',(1.04872505851243,-0.26577216648544,10.3597071335657));
#11801=CARTESIAN_POINT('Ctrl Pts',(1.07750116603121,0.243190015038482,10.3835038803323));
#11802=CARTESIAN_POINT('Ctrl Pts',(0.781688530878207,0.777999980609408,
10.4120173608425));
#11803=CARTESIAN_POINT('Ctrl Pts',(0.247719136142376,1.07295015546241,10.4404872688827));
#11804=CARTESIAN_POINT('Ctrl Pts',(-0.360486616831365,1.03867188015668,
10.4689126947258));
#11805=CARTESIAN_POINT('Ctrl Pts',(-0.856395421979649,0.686612064758622,
10.4972927514314));
#11806=CARTESIAN_POINT('Ctrl Pts',(-1.08862861454113,0.125592182065228,
10.5256265935356));
#11807=CARTESIAN_POINT('Ctrl Pts',(-0.986944606168628,-0.472001059894419,
10.5539134034074));
#11808=CARTESIAN_POINT('Ctrl Pts',(-0.583594151562567,-0.923132799570535,
10.5821523997639));
#11809=CARTESIAN_POINT('Ctrl Pts',(-0.00304950196324622,-1.09023227406354,
10.6103428416619));
#11810=CARTESIAN_POINT('Ctrl Pts',(0.576397100829433,-0.923141572582211,
10.6384840153271));
#11811=CARTESIAN_POINT('Ctrl Pts',(0.977415745977647,-0.474174920735025,
10.666575250779));
#11812=CARTESIAN_POINT('Ctrl Pts',(1.07791854333959,0.118262177227866,10.6946159100158));
#11813=CARTESIAN_POINT('Ctrl Pts',(0.848237687346995,0.672348815808936,
10.7226053954193));
#11814=CARTESIAN_POINT('Ctrl Pts',(0.35987034323251,1.01866632704243,10.750543145368));
#11815=CARTESIAN_POINT('Ctrl Pts',(-0.23677931351889,1.05200727853759,10.7784286311663));
#11816=CARTESIAN_POINT('Ctrl Pts',(-0.758730842080508,0.763346883548158,
10.8062613781485));
#11817=CARTESIAN_POINT('Ctrl Pts',(-1.04655744183574,0.242222537004657,
10.8340409125563));
#11818=CARTESIAN_POINT('Ctrl Pts',(-1.01308793288556,-0.351003613269005,
10.8617668734456));
#11819=CARTESIAN_POINT('Ctrl Pts',(-0.669814425530371,-0.834593746223134,
10.889438771651));
#11820=CARTESIAN_POINT('Ctrl Pts',(-0.122977155730889,-1.06092281666227,
10.9170565165848));
#11821=CARTESIAN_POINT('Ctrl Pts',(0.459284142389985,-0.962004532278344,
10.9446192376113));
#11822=CARTESIAN_POINT('Ctrl Pts',(0.898703292351648,-0.568910379520766,
10.9721279252064));
#11823=CARTESIAN_POINT('Ctrl Pts',(1.0071027576084,-0.192548907318078,10.9904290025552));
#11824=CARTESIAN_POINT('Ctrl Pts',(1.00712819276269,-0.00361011030918905,
10.999573158519));
#11825=CARTESIAN_POINT('Origin',(1.,-2.44249065417534E-15,10.925));
#11826=CARTESIAN_POINT('Origin',(1.,-2.44249065417534E-15,10.925));
#11827=CARTESIAN_POINT('Origin',(1.,0.,7.875));
#13204=UNCERTAINTY_MEASURE_WITH_UNIT(LENGTH_MEASURE(0.001),#13278,
'DISTANCE_ACCURACY_VALUE',
'Maximum model space distance between geometric entities at asserted c
onnectivities');
#13233=UNCERTAINTY_MEASURE_WITH_UNIT(LENGTH_MEASURE(0.001),#13278,
'DISTANCE_ACCURACY_VALUE',
'Maximum model space distance between geometric entities at asserted c
onnectivities');
#13248=(
GEOMETRIC_REPRESENTATION_CONTEXT(3)
GLOBAL_UNCERTAINTY_ASSIGNED_CONTEXT((#13204))
GLOBAL_UNIT_ASSIGNED_CONTEXT((#13278,#13280,#13281))
REPRESENTATION_CONTEXT('','3D')
);
#13277=(
GEOMETRIC_REPRESENTATION_CONTEXT(3)
GLOBAL_UNCERTAINTY_ASSIGNED_CONTEXT((#13233))
GLOBAL_UNIT_ASSIGNED_CONTEXT((#13278,#13280,#13281))
REPRESENTATION_CONTEXT('','3D')
);
#13278=(
LENGTH_UNIT()
NAMED_UNIT(*)
SI_UNIT(.CENTI.,.METRE.)
);
#13280=(
NAMED_UNIT(*)
PLANE_ANGLE_UNIT()
SI_UNIT($,.RADIAN.)
);
#13281=(
NAMED_UNIT(*)
SI_UNIT($,.STERADIAN.)
SOLID_ANGLE_UNIT()
);
#13296=SHAPE_DEFINITION_REPRESENTATION(#13339,#13453);
#13339=PRODUCT_DEFINITION_SHAPE('',$,#13497);
#13453=SHAPE_REPRESENTATION('',(#7149),#13248);
#13482=PRODUCT_DEFINITION_CONTEXT('part definition',#13613,'design');
#13497=PRODUCT_DEFINITION('Installed return spring',
'Installed return spring',#13540,#13482);
#13540=PRODUCT_DEFINITION_FORMATION('',$,#13629);
#13613=APPLICATION_CONTEXT(
'Core Data for Automotive Mechanical Design Process');
#13614=PRODUCT_CONTEXT('part definition',#13613,'mechanical');
#13629=PRODUCT('Installed return spring','Installed return spring',
'Installed return spring',(#13614));
#13714=COLOUR_RGB('Grey',0.48,0.52,0.57);
#13715=FILL_AREA_STYLE_COLOUR('',#13714);
#13716=FILL_AREA_STYLE('',(#13715));
#13717=SURFACE_STYLE_FILL_AREA(#13716);
#13718=SURFACE_SIDE_STYLE('',(#13717));
#13719=SURFACE_STYLE_USAGE(.BOTH.,#13718);
#13720=PRESENTATION_STYLE_ASSIGNMENT((#13719));
ENDSEC;
END-ISO-10303-21;
